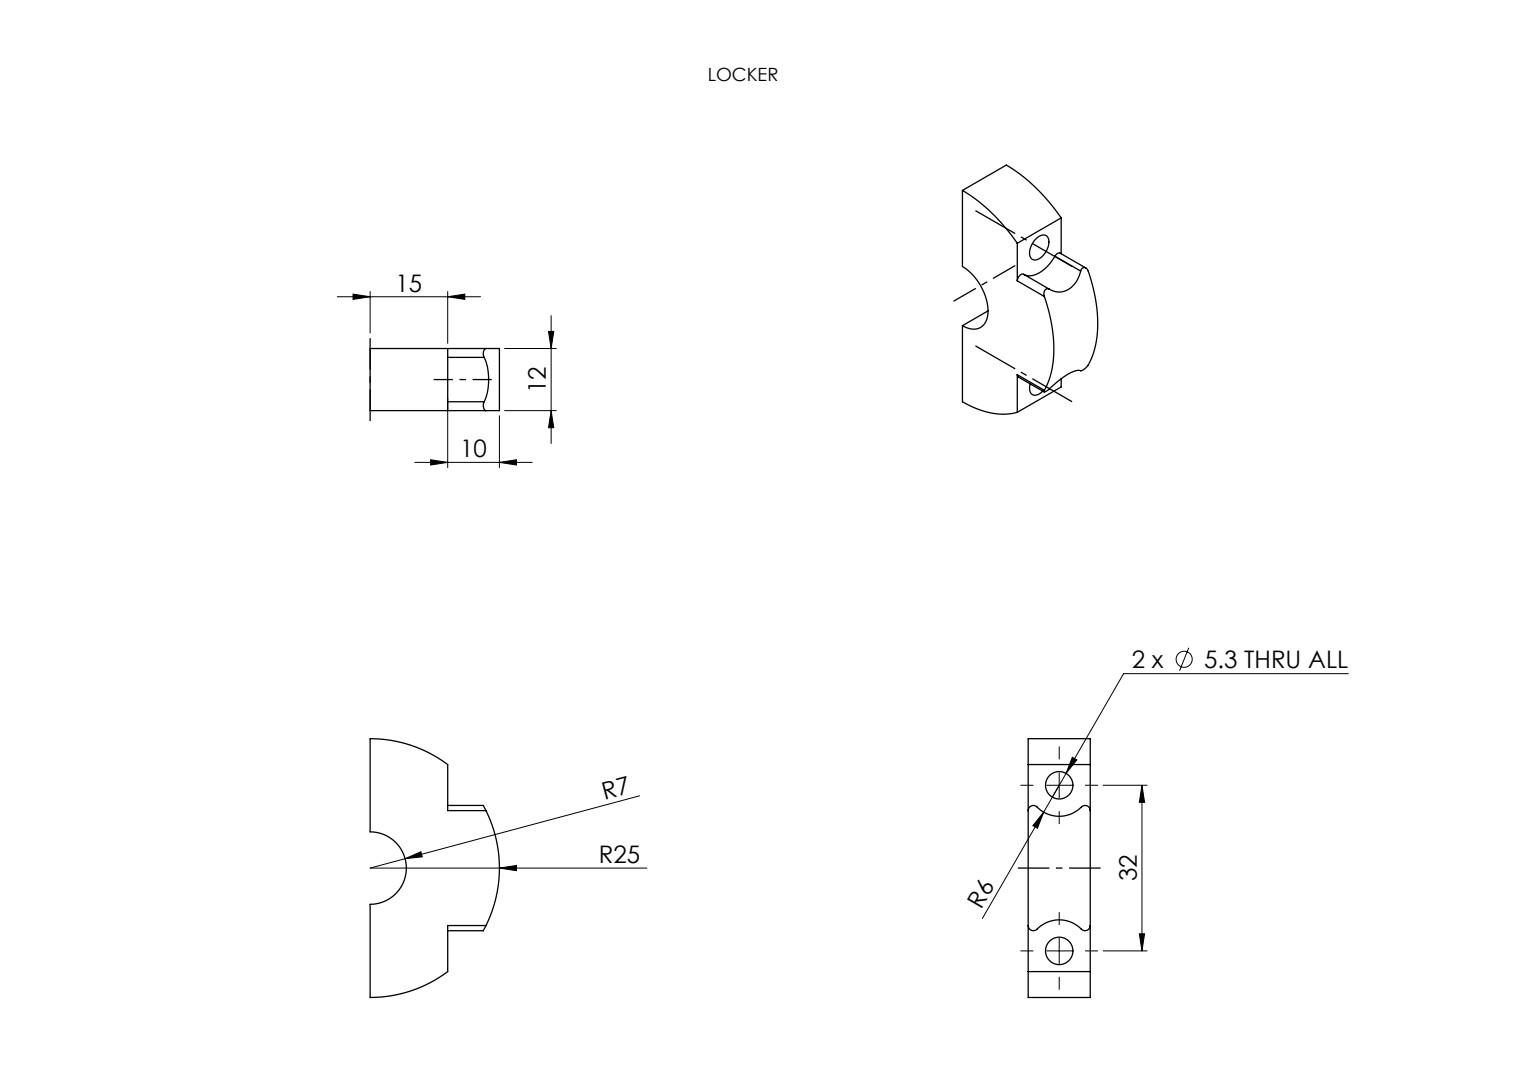
ISO-10303-21;
HEADER;
FILE_DESCRIPTION (('STEP AP214'),
    '1' );
FILE_NAME ('locker.step',
    '2026-10-08T14:09:18',
    ( '' ),
    ( '' ),
    'SwSTEP 2.0',
    'SolidWorks 2026',
    '' );
FILE_SCHEMA (( 'AUTOMOTIVE_DESIGN' ));
ENDSEC;

DATA;
#1=LINE ( 'NONE', #1937, #4329 ) ;
#6=AXIS2_PLACEMENT_3D ( 'NONE', #3174, #4687, #3807 ) ;
#21=AXIS2_PLACEMENT_3D ( 'NONE', #885, #4593, #1214 ) ;
#23=ORIENTED_EDGE ( 'NONE', *, *, #1515, .T. ) ;
#25=CARTESIAN_POINT ( 'NONE',  ( 22.89074894326665088, 10.05057747304974924, -26.80355754512474675 ) ) ;
#32=CARTESIAN_POINT ( 'NONE',  ( 15.00000000000000178, -16.00000000000000000, -26.00000000000000355 ) ) ;
#39=DIRECTION ( 'NONE',  ( 0.000000000000000000, 0.000000000000000000, -1.000000000000000000 ) ) ;
#60=ORIENTED_EDGE ( 'NONE', *, *, #3152, .T. ) ;
#64=DIRECTION ( 'NONE',  ( 0.000000000000000000, -1.000000000000000000, 0.000000000000000000 ) ) ;
#67=CARTESIAN_POINT ( 'NONE',  ( 25.00000000000000000, -11.80087472665741011, -21.71428571428571530 ) ) ;
#72=CARTESIAN_POINT ( 'NONE',  ( 22.90859662698202470, -10.00982993400317334, -25.60100662543646877 ) ) ;
#79=DIRECTION ( 'NONE',  ( 1.000000000000000000, 0.000000000000000000, 0.000000000000000000 ) ) ;
#81=CARTESIAN_POINT ( 'NONE',  ( 21.90226041726126383, 12.05376714070078847, -31.32044994803182547 ) ) ;
#88=CARTESIAN_POINT ( 'NONE',  ( 15.00000000000000000, 11.10102051443364424, -21.00000000000000000 ) ) ;
#101=AXIS2_PLACEMENT_3D ( 'NONE', #4841, #1750, #2213 ) ;
#104=CARTESIAN_POINT ( 'NONE',  ( 22.03949535914419755, -11.80087472665740655, -21.71428571428571885 ) ) ;
#113=EDGE_CURVE ( 'NONE', #181, #2456, #4183, .T. ) ;
#114=ORIENTED_EDGE ( 'NONE', *, *, #457, .T. ) ;
#122=CIRCLE ( 'NONE', #3524, 2.649999999999995914 ) ;
#129=EDGE_LOOP ( 'NONE', ( #232, #1337, #3287, #640, #1099, #3548 ) ) ;
#133=EDGE_CURVE ( 'NONE', #4849, #2456, #528, .T. ) ;
#139=SURFACE_STYLE_USAGE ( .BOTH. , #2050 ) ;
#141=CYLINDRICAL_SURFACE ( 'NONE', #2344, 2.649999999999992806 ) ;
#145=CARTESIAN_POINT ( 'NONE',  ( 25.00000000000000000, 11.80087472665740478, -30.28571428571428470 ) ) ;
#155=CARTESIAN_POINT ( 'NONE',  ( 15.00000000000000000, 16.00000000000000000, -26.00000000000000355 ) ) ;
#156=CARTESIAN_POINT ( 'NONE',  ( 22.03949535914419755, -11.80087472665740655, -21.71428571428571885 ) ) ;
#159=B_SPLINE_CURVE_WITH_KNOTS ( 'NONE', 3,
 ( #3123, #2291, #1168, #2640, #4187, #3835, #3809, #759, #1888, #81, #4617, #385, #2749, #3439, #2697, #3415 ),
 .UNSPECIFIED., .F., .F.,
 ( 4, 2, 2, 2, 2, 2, 2, 4 ),
 ( 0.000000000000000000, 0.0003092645584586380158, 0.0006185291169172760315, 0.0009277936753759139388, 0.001237058233834552063, 0.001546322792293189970, 0.001855587350751827878, 0.002474116467669114968 ),
 .UNSPECIFIED. ) ;
#160=ORIENTED_EDGE ( 'NONE', *, *, #457, .F. ) ;
#162=CARTESIAN_POINT ( 'NONE',  ( 22.40016391766193138, 11.10102051443364424, -20.00000000000000000 ) ) ;
#165=VERTEX_POINT ( 'NONE', #2693 ) ;
#180=ORIENTED_EDGE ( 'NONE', *, *, #1366, .T. ) ;
#181=VERTEX_POINT ( 'NONE', #4357 ) ;
#184=AXIS2_PLACEMENT_3D ( 'NONE', #4270, #4673, #3105 ) ;
#190=B_SPLINE_CURVE_WITH_KNOTS ( 'NONE', 3,
 ( #2928, #244, #278, #4394, #4375, #967, #201, #1739, #4801, #3276 ),
 .UNSPECIFIED., .F., .F.,
 ( 4, 2, 2, 2, 4 ),
 ( 0.000000000000000000, 0.0006190800217238748033, 0.001238160043447749607, 0.001857240065171624410, 0.002476320086895499213 ),
 .UNSPECIFIED. ) ;
#191=VECTOR ( 'NONE', #2924, 1000.000000000000000 ) ;
#193=SURFACE_STYLE_FILL_AREA ( #525 ) ;
#201=CARTESIAN_POINT ( 'NONE',  ( 22.04417985544613146, -11.79351823160729751, -31.74594383812769749 ) ) ;
#213=CARTESIAN_POINT ( 'NONE',  ( 0.000000000000000000, -25.00000000000000000, -20.00000000000000000 ) ) ;
#221=CARTESIAN_POINT ( 'NONE',  ( 25.00000000000000000, 11.10102051443364424, -21.00000000000000000 ) ) ;
#229=CARTESIAN_POINT ( 'NONE',  ( 0.000000000000000000, 0.000000000000000000, -32.00000000000000000 ) ) ;
#230=FACE_OUTER_BOUND ( 'NONE', #3929, .T. ) ;
#232=ORIENTED_EDGE ( 'NONE', *, *, #1612, .F. ) ;
#244=CARTESIAN_POINT ( 'NONE',  ( 21.96482728828171460, -11.94032596560094461, -30.42234803747852467 ) ) ;
#260=DIRECTION ( 'NONE',  ( 1.000000000000000000, -0.000000000000000000, -0.000000000000000000 ) ) ;
#263=PRODUCT ( 'locker', 'locker', '', ( #3647 ) ) ;
#266=VECTOR ( 'NONE', #64, 1000.000000000000000 ) ;
#268=CIRCLE ( 'NONE', #3072, 25.00000000000000000 ) ;
#273=ORIENTED_EDGE ( 'NONE', *, *, #2286, .F. ) ;
#278=CARTESIAN_POINT ( 'NONE',  ( 21.90877321452243365, -12.04191644460182431, -30.60336459293191780 ) ) ;
#284=CARTESIAN_POINT ( 'NONE',  ( 22.76747806470418567, 10.32821797429375010, -24.00231280675427215 ) ) ;
#294=DIRECTION ( 'NONE',  ( 0.000000000000000000, 0.000000000000000000, -1.000000000000000000 ) ) ;
#295=ADVANCED_FACE ( 'NONE', ( #2885 ), #673, .T. ) ;
#298=B_SPLINE_CURVE_WITH_KNOTS ( 'NONE', 3,
 ( #2171, #3292, #3229, #3661, #2073, #4458, #3590, #4061, #2542, #162 ),
 .UNSPECIFIED., .F., .F.,
 ( 4, 2, 2, 2, 4 ),
 ( 0.000000000000000000, 0.0006190800217238756707, 0.001238160043447751341, 0.001857240065171627012, 0.002476320086895502683 ),
 .UNSPECIFIED. ) ;
#307=DIRECTION ( 'NONE',  ( 0.000000000000000000, 0.000000000000000000, -1.000000000000000000 ) ) ;
#310=DIRECTION ( 'NONE',  ( 0.000000000000000000, 1.000000000000000000, 0.000000000000000000 ) ) ;
#318=VERTEX_POINT ( 'NONE', #4781 ) ;
#343=MECHANICAL_DESIGN_GEOMETRIC_PRESENTATION_REPRESENTATION('',(#3776),#4337);
#347=( NAMED_UNIT ( * ) PLANE_ANGLE_UNIT ( ) SI_UNIT ( $, .RADIAN. ) );
#364=DIRECTION ( 'NONE',  ( 0.000000000000000000, 0.000000000000000000, -1.000000000000000000 ) ) ;
#371=ORIENTED_EDGE ( 'NONE', *, *, #1787, .F. ) ;
#375=CARTESIAN_POINT ( 'NONE',  ( 22.61674500023159240, -10.65336738338371347, -28.73004557699725936 ) ) ;
#376=PLANE ( 'NONE',  #1226 ) ;
#381=ADVANCED_FACE ( 'NONE', ( #1705 ), #3239, .T. ) ;
#385=CARTESIAN_POINT ( 'NONE',  ( 21.87320774003120150, 12.10631999347636167, -31.01543084472370992 ) ) ;
#390=LINE ( 'NONE', #1915, #2331 ) ;
#393=UNCERTAINTY_MEASURE_WITH_UNIT (LENGTH_MEASURE( 1.000000000000000082E-05 ), #500, 'distance_accuracy_value', 'NONE');
#394=CARTESIAN_POINT ( 'NONE',  ( 15.00000000000000000, 11.10102051443364424, -20.00000000000000000 ) ) ;
#395=CARTESIAN_POINT ( 'NONE',  ( -3.642919299551294898E-14, -16.00000000000000000, -26.00000000000000355 ) ) ;
#400=EDGE_CURVE ( 'NONE', #2569, #4849, #4958, .T. ) ;
#402=DIRECTION ( 'NONE',  ( 1.000000000000000000, 2.036697447658493800E-15, 0.000000000000000000 ) ) ;
#427=CIRCLE ( 'NONE', #3306, 2.649999999999985700 ) ;
#429=CARTESIAN_POINT ( 'NONE',  ( 0.000000000000000000, 0.000000000000000000, -32.00000000000000000 ) ) ;
#437=CARTESIAN_POINT ( 'NONE',  ( 22.66008913276283820, 10.56067522606771547, -28.54043899563736986 ) ) ;
#457=EDGE_CURVE ( 'NONE', #181, #2569, #122, .T. ) ;
#464=CARTESIAN_POINT ( 'NONE',  ( 22.88998946896871445, 10.05230818559221539, -25.18361442742383360 ) ) ;
#472=CARTESIAN_POINT ( 'NONE',  ( 21.87533763385574659, -12.10248395817102107, -21.08882388928228835 ) ) ;
#485=PRODUCT_DEFINITION_CONTEXT ( 'detailed design', #2667, 'design' ) ;
#486=CARTESIAN_POINT ( 'NONE',  ( 22.31344532614783205, -11.27701289969359522, -22.27898711539451071 ) ) ;
#489=EDGE_CURVE ( 'NONE', #3217, #2692, #1229, .T. ) ;
#492=SHAPE_DEFINITION_REPRESENTATION ( #1211, #4221 ) ;
#500=( LENGTH_UNIT ( ) NAMED_UNIT ( * ) SI_UNIT ( .MILLI., .METRE. ) );
#503=AXIS2_PLACEMENT_3D ( 'NONE', #890, #2321, #39 ) ;
#510=VECTOR ( 'NONE', #740, 1000.000000000000000 ) ;
#512=ORIENTED_EDGE ( 'NONE', *, *, #1917, .T. ) ;
#516=DIRECTION ( 'NONE',  ( 1.000000000000000000, -0.000000000000000000, -0.000000000000000000 ) ) ;
#522=DIRECTION ( 'NONE',  ( 1.000000000000000000, -0.000000000000000000, -0.000000000000000000 ) ) ;
#525=FILL_AREA_STYLE ('',( #2096 ) ) ;
#528=CIRCLE ( 'NONE', #4589, 2.649999999999985700 ) ;
#563=ORIENTED_EDGE ( 'NONE', *, *, #3713, .T. ) ;
#580=COLOUR_RGB ( '', 0.72549020, 0.75294118, 0.79215686) ;
#586=VERTEX_POINT ( 'NONE', #1997 ) ;
#588=DIRECTION ( 'NONE',  ( 0.000000000000000000, 0.000000000000000000, 1.000000000000000000 ) ) ;
#599=DIRECTION ( 'NONE',  ( -1.000000000000000000, 0.000000000000000000, 0.000000000000000000 ) ) ;
#603=DIRECTION ( 'NONE',  ( -1.000000000000000000, 0.000000000000000000, 0.000000000000000000 ) ) ;
#604=CARTESIAN_POINT ( 'NONE',  ( 15.00000000000000000, -11.80087472665740655, -21.71428571428571885 ) ) ;
#612=EDGE_LOOP ( 'NONE', ( #60, #1655 ) ) ;
#617=MECHANICAL_DESIGN_GEOMETRIC_PRESENTATION_REPRESENTATION('',(#1267),#2875);
#618=DIRECTION ( 'NONE',  ( -0.000000000000000000, -0.000000000000000000, 1.000000000000000000 ) ) ;
#620=PRESENTATION_STYLE_ASSIGNMENT (( #4050 ) ) ;
#628=EDGE_CURVE ( 'NONE', #4218, #3494, #3207, .T. ) ;
#636=FACE_BOUND ( 'NONE', #612, .T. ) ;
#640=ORIENTED_EDGE ( 'NONE', *, *, #4116, .T. ) ;
#649=CYLINDRICAL_SURFACE ( 'NONE', #973, 6.999999999999999112 ) ;
#651=CIRCLE ( 'NONE', #978, 2.649999999999995914 ) ;
#668=DIRECTION ( 'NONE',  ( 1.000000000000000000, 0.000000000000000000, 0.000000000000000000 ) ) ;
#672=CARTESIAN_POINT ( 'NONE',  ( 0.000000000000000000, -25.00000000000000000, -32.00000000000000000 ) ) ;
#673=CYLINDRICAL_SURFACE ( 'NONE', #4506, 1.000000000000000888 ) ;
#684=EDGE_CURVE ( 'NONE', #2597, #4218, #190, .T. ) ;
#688=LINE ( 'NONE', #3368, #510 ) ;
#693=ORIENTED_EDGE ( 'NONE', *, *, #4446, .T. ) ;
#696=CARTESIAN_POINT ( 'NONE',  ( 0.000000000000000000, 0.000000000000000000, -20.00000000000000000 ) ) ;
#698=CARTESIAN_POINT ( 'NONE',  ( 2.444036937190193033E-14, 6.999999999999999112, -20.00000000000000000 ) ) ;
#699=FACE_BOUND ( 'NONE', #2377, .T. ) ;
#705=CARTESIAN_POINT ( 'NONE',  ( 0.000000000000000000, 25.00000000000000000, -32.00000000000000000 ) ) ;
#710=DIRECTION ( 'NONE',  ( 0.000000000000000000, 0.000000000000000000, 1.000000000000000000 ) ) ;
#719=ADVANCED_FACE ( 'NONE', ( #2078 ), #1718, .F. ) ;
#730=DIRECTION ( 'NONE',  ( 0.000000000000000000, 0.000000000000000000, -1.000000000000000000 ) ) ;
#740=DIRECTION ( 'NONE',  ( -2.036697447658493800E-15, 1.000000000000000000, 0.000000000000000000 ) ) ;
#746=EDGE_CURVE ( 'NONE', #2092, #2240, #994, .T. ) ;
#748=CARTESIAN_POINT ( 'NONE',  ( 22.31144310522464735, -11.28096319364321509, -29.72586080439007006 ) ) ;
#749=EDGE_CURVE ( 'NONE', #1695, #3657, #3997, .T. ) ;
#755=ADVANCED_BREP_SHAPE_REPRESENTATION ( '', ( #2079, #1918 ), #1581 ) ;
#759=CARTESIAN_POINT ( 'NONE',  ( 21.97815564317848924, 11.91494984865602191, -31.58906108478248953 ) ) ;
#781=CARTESIAN_POINT ( 'NONE',  ( 22.04753367391286645, -11.78607713658132994, -20.26503649943386876 ) ) ;
#787=FILL_AREA_STYLE ('',( #1511 ) ) ;
#796=VECTOR ( 'NONE', #2151, 1000.000000000000000 ) ;
#797=CARTESIAN_POINT ( 'NONE',  ( 22.87614623887219167, 10.08384657499285808, -24.98007506026046798 ) ) ;
#801=AXIS2_PLACEMENT_3D ( 'NONE', #2152, #4779, #1345 ) ;
#807=CARTESIAN_POINT ( 'NONE',  ( 21.88691174701116182, -12.08152700620045117, -20.77757659040560512 ) ) ;
#810=CIRCLE ( 'NONE', #1521, 2.649999999999985700 ) ;
#821=ORIENTED_EDGE ( 'NONE', *, *, #3902, .T. ) ;
#827=ORIENTED_EDGE ( 'NONE', *, *, #2659, .T. ) ;
#831=CARTESIAN_POINT ( 'NONE',  ( 22.91733099102425442, 9.989778831080645460, -25.99421712970024245 ) ) ;
#833=DIRECTION ( 'NONE',  ( 0.000000000000000000, 0.000000000000000000, 1.000000000000000000 ) ) ;
#839=LINE ( 'NONE', #2341, #3531 ) ;
#840=CARTESIAN_POINT ( 'NONE',  ( 21.87320774003119794, -12.10631999347636345, -20.98456915527629363 ) ) ;
#847=ORIENTED_EDGE ( 'NONE', *, *, #133, .T. ) ;
#849=EDGE_CURVE ( 'NONE', #1731, #4866, #1094, .T. ) ;
#855=CARTESIAN_POINT ( 'NONE',  ( 22.52717933085839874, -10.84147272832753472, -22.92928814334748466 ) ) ;
#862=FACE_OUTER_BOUND ( 'NONE', #1009, .T. ) ;
#864=ORIENTED_EDGE ( 'NONE', *, *, #3599, .F. ) ;
#870=EDGE_CURVE ( 'NONE', #2692, #3603, #4723, .T. ) ;
#878=CARTESIAN_POINT ( 'NONE',  ( 15.00000000000000000, -11.10102051443364068, -32.00000000000000000 ) ) ;
#880=EDGE_CURVE ( 'NONE', #3891, #4613, #1042, .T. ) ;
#882=AXIS2_PLACEMENT_3D ( 'NONE', #3346, #4515, #1738 ) ;
#884=DIRECTION ( 'NONE',  ( 0.000000000000000000, 0.000000000000000000, -1.000000000000000000 ) ) ;
#885=CARTESIAN_POINT ( 'NONE',  ( 25.00000000000000000, -11.10102051443364424, -21.00000000000000000 ) ) ;
#890=CARTESIAN_POINT ( 'NONE',  ( 15.00000000000000000, 11.10102051443364068, -31.00000000000000000 ) ) ;
#892=AXIS2_PLACEMENT_3D ( 'NONE', #2942, #989, #2146 ) ;
#916=DIRECTION ( 'NONE',  ( 0.000000000000000000, 0.000000000000000000, -1.000000000000000000 ) ) ;
#918=CARTESIAN_POINT ( 'NONE',  ( 25.00000000000000000, 11.10102051443364068, -31.00000000000000000 ) ) ;
#924=VECTOR ( 'NONE', #3089, 1000.000000000000000 ) ;
#929=ORIENTED_EDGE ( 'NONE', *, *, #746, .F. ) ;
#932=LINE ( 'NONE', #3978, #3232 ) ;
#935=CARTESIAN_POINT ( 'NONE',  ( 0.000000000000000000, 0.000000000000000000, -20.00000000000000000 ) ) ;
#942=LINE ( 'NONE', #213, #4561 ) ;
#943=CARTESIAN_POINT ( 'NONE',  ( 25.00000000000000000, 0.000000000000000000, -20.00000000000000000 ) ) ;
#959=ORIENTED_EDGE ( 'NONE', *, *, #3343, .T. ) ;
#963=EDGE_CURVE ( 'NONE', #1731, #3126, #1842, .T. ) ;
#965=DIRECTION ( 'NONE',  ( 1.000000000000000000, 0.000000000000000000, 0.000000000000000000 ) ) ;
#966=EDGE_CURVE ( 'NONE', #4690, #2597, #390, .T. ) ;
#967=CARTESIAN_POINT ( 'NONE',  ( 21.97031423931356287, -11.92955703141274881, -31.59565500209243183 ) ) ;
#973=AXIS2_PLACEMENT_3D ( 'NONE', #3359, #2664, #1028 ) ;
#978=AXIS2_PLACEMENT_3D ( 'NONE', #2150, #2475, #2105 ) ;
#985=ORIENTED_EDGE ( 'NONE', *, *, #2110, .T. ) ;
#987=VERTEX_POINT ( 'NONE', #1248 ) ;
#989=DIRECTION ( 'NONE',  ( 1.000000000000000000, -0.000000000000000000, -0.000000000000000000 ) ) ;
#992=CARTESIAN_POINT ( 'NONE',  ( 15.00000000000000000, -20.00000000000000355, -32.00000000000000000 ) ) ;
#994=LINE ( 'NONE', #2477, #4000 ) ;
#1009=EDGE_LOOP ( 'NONE', ( #3602, #4092, #2424, #2514 ) ) ;
#1024=VERTEX_POINT ( 'NONE', #4598 ) ;
#1026=CARTESIAN_POINT ( 'NONE',  ( 22.52496067886514197, 10.84608396733234592, -22.92156229269478374 ) ) ;
#1028=DIRECTION ( 'NONE',  ( 1.000000000000000000, 0.000000000000000000, 0.000000000000000000 ) ) ;
#1036=ORIENTED_EDGE ( 'NONE', *, *, #4737, .T. ) ;
#1042=LINE ( 'NONE', #3766, #4728 ) ;
#1060=EDGE_CURVE ( 'NONE', #3126, #4359, #2094, .T. ) ;
#1067=VERTEX_POINT ( 'NONE', #1221 ) ;
#1069=CARTESIAN_POINT ( 'NONE',  ( 22.03949535914419755, -11.80087472665740655, -21.71428571428571885 ) ) ;
#1081=CARTESIAN_POINT ( 'NONE',  ( 22.40016391766193493, 11.10102051443364068, -32.00000000000000000 ) ) ;
#1094=LINE ( 'NONE', #3399, #2408 ) ;
#1096=ORIENTED_EDGE ( 'NONE', *, *, #3247, .T. ) ;
#1099=ORIENTED_EDGE ( 'NONE', *, *, #1951, .F. ) ;
#1115=DIRECTION ( 'NONE',  ( 1.000000000000000000, 0.000000000000000000, 0.000000000000000000 ) ) ;
#1143=VECTOR ( 'NONE', #4180, 1000.000000000000000 ) ;
#1145=FACE_OUTER_BOUND ( 'NONE', #2865, .T. ) ;
#1146=CARTESIAN_POINT ( 'NONE',  ( 0.000000000000000000, 0.000000000000000000, 0.000000000000000000 ) ) ;
#1147=CARTESIAN_POINT ( 'NONE',  ( 15.00000000000000000, 16.00000000000000000, -26.00000000000000355 ) ) ;
#1158=CARTESIAN_POINT ( 'NONE',  ( 22.76902711785762534, -10.32479573876449486, -24.01193718893786411 ) ) ;
#1163=EDGE_LOOP ( 'NONE', ( #929, #3191, #2786, #3592, #1633, #1962 ) ) ;
#1164=DIRECTION ( 'NONE',  ( 1.000000000000000000, -0.000000000000000000, -0.000000000000000000 ) ) ;
#1168=CARTESIAN_POINT ( 'NONE',  ( 22.30769810302473388, 11.28612666381332730, -31.98709346889334881 ) ) ;
#1174=ORIENTED_EDGE ( 'NONE', *, *, #4886, .F. ) ;
#1192=CARTESIAN_POINT ( 'NONE',  ( 22.21646894734064759, -11.46466559648295558, -20.06384827235568835 ) ) ;
#1206=CARTESIAN_POINT ( 'NONE',  ( 22.18526740102420547, -11.52862861652370441, -30.01896866400023356 ) ) ;
#1211=PRODUCT_DEFINITION_SHAPE ( 'NONE', 'NONE',  #2072 ) ;
#1214=DIRECTION ( 'NONE',  ( 0.000000000000000000, 0.000000000000000000, 1.000000000000000000 ) ) ;
#1219=( NAMED_UNIT ( * ) SI_UNIT ( $, .STERADIAN. ) SOLID_ANGLE_UNIT ( ) );
#1221=CARTESIAN_POINT ( 'NONE',  ( 0.000000000000000000, 25.00000000000000000, -32.00000000000000000 ) ) ;
#1224=LINE ( 'NONE', #3520, #266 ) ;
#1225=EDGE_LOOP ( 'NONE', ( #3596, #4059, #4019, #985 ) ) ;
#1226=AXIS2_PLACEMENT_3D ( 'NONE', #1449, #402, #1496 ) ;
#1229=LINE ( 'NONE', #67, #4473 ) ;
#1230=AXIS2_PLACEMENT_3D ( 'NONE', #88, #1590, #4909 ) ;
#1232=ORIENTED_EDGE ( 'NONE', *, *, #1612, .T. ) ;
#1234=CARTESIAN_POINT ( 'NONE',  ( 22.66008913276283110, -10.56067522606771547, -23.45956100436263725 ) ) ;
#1241=DIRECTION ( 'NONE',  ( 1.000000000000000000, -0.000000000000000000, -0.000000000000000000 ) ) ;
#1242=EDGE_CURVE ( 'NONE', #2366, #165, #942, .T. ) ;
#1247=ORIENTED_EDGE ( 'NONE', *, *, #1242, .T. ) ;
#1248=CARTESIAN_POINT ( 'NONE',  ( 6.999999999999999112, 0.000000000000000000, -32.00000000000000000 ) ) ;
#1258=EDGE_LOOP ( 'NONE', ( #1815, #3183, #2999, #3488 ) ) ;
#1267=STYLED_ITEM ( 'NONE', ( #1990 ), #755 ) ;
#1269=( NAMED_UNIT ( * ) PLANE_ANGLE_UNIT ( ) SI_UNIT ( $, .RADIAN. ) );
#1274=CYLINDRICAL_SURFACE ( 'NONE', #4467, 25.00000000000000000 ) ;
#1276=ORIENTED_EDGE ( 'NONE', *, *, #4303, .T. ) ;
#1286=DIRECTION ( 'NONE',  ( -1.000000000000000000, 0.000000000000000000, 0.000000000000000000 ) ) ;
#1297=CIRCLE ( 'NONE', #3372, 25.00000000000000000 ) ;
#1300=AXIS2_PLACEMENT_3D ( 'NONE', #229, #4403, #603 ) ;
#1303=CIRCLE ( 'NONE', #2022, 2.649999999999995914 ) ;
#1307=VECTOR ( 'NONE', #2791, 1000.000000000000000 ) ;
#1312=EDGE_LOOP ( 'NONE', ( #3317, #1232, #2731, #3928, #2819, #959, #2054, #4784, #3946, #4335, #3757, #4091 ) ) ;
#1322=FACE_OUTER_BOUND ( 'NONE', #2719, .T. ) ;
#1337=ORIENTED_EDGE ( 'NONE', *, *, #746, .T. ) ;
#1345=DIRECTION ( 'NONE',  ( 0.000000000000000000, 0.000000000000000000, -1.000000000000000000 ) ) ;
#1366=EDGE_CURVE ( 'NONE', #4359, #318, #4531, .T. ) ;
#1370=LINE ( 'NONE', #672, #4067 ) ;
#1396=EDGE_CURVE ( 'NONE', #586, #3657, #2656, .T. ) ;
#1408=CYLINDRICAL_SURFACE ( 'NONE', #3219, 1.000000000000000888 ) ;
#1413=DIRECTION ( 'NONE',  ( 1.000000000000000000, 0.000000000000000000, 0.000000000000000000 ) ) ;
#1424=LINE ( 'NONE', #3707, #2981 ) ;
#1434=DIRECTION ( 'NONE',  ( -1.000000000000000000, -0.000000000000000000, -0.000000000000000000 ) ) ;
#1445=ADVANCED_FACE ( 'NONE', ( #2672 ), #1481, .F. ) ;
#1446=CIRCLE ( 'NONE', #1300, 6.999999999999999112 ) ;
#1449=CARTESIAN_POINT ( 'NONE',  ( 0.000000000000000000, -25.00000000000000000, -32.00000000000000000 ) ) ;
#1466=CARTESIAN_POINT ( 'NONE',  ( 25.00000000000000000, 0.000000000000000000, -32.00000000000000000 ) ) ;
#1472=ORIENTED_EDGE ( 'NONE', *, *, #4303, .F. ) ;
#1475=FACE_OUTER_BOUND ( 'NONE', #3274, .T. ) ;
#1478=EDGE_CURVE ( 'NONE', #1067, #318, #1297, .T. ) ;
#1481=PLANE ( 'NONE',  #2574 ) ;
#1490=UNCERTAINTY_MEASURE_WITH_UNIT (LENGTH_MEASURE( 1.000000000000000082E-05 ), #4932, 'distance_accuracy_value', 'NONE');
#1496=DIRECTION ( 'NONE',  ( -2.036697447658493800E-15, 1.000000000000000000, 0.000000000000000000 ) ) ;
#1508=ADVANCED_FACE ( 'NONE', ( #3912 ), #3833, .F. ) ;
#1511=FILL_AREA_STYLE_COLOUR ( '', #580 ) ;
#1515=EDGE_CURVE ( 'NONE', #318, #4003, #1, .T. ) ;
#1521=AXIS2_PLACEMENT_3D ( 'NONE', #32, #1241, #3099 ) ;
#1534=CARTESIAN_POINT ( 'NONE',  ( 22.40016391766193138, -11.10102051443364424, -20.00000000000000000 ) ) ;
#1535=ORIENTED_EDGE ( 'NONE', *, *, #3247, .F. ) ;
#1539=EDGE_LOOP ( 'NONE', ( #3461, #1174, #3112, #4718 ) ) ;
#1544=EDGE_CURVE ( 'NONE', #2456, #4849, #810, .T. ) ;
#1554=CARTESIAN_POINT ( 'NONE',  ( 22.47483654244695472, -10.94974330264383156, -29.24541893584931529 ) ) ;
#1573=CARTESIAN_POINT ( 'NONE',  ( 22.03949535914419755, -11.80087472665740478, -30.28571428571428470 ) ) ;
#1581=( GEOMETRIC_REPRESENTATION_CONTEXT ( 3 ) GLOBAL_UNCERTAINTY_ASSIGNED_CONTEXT ( ( #393 ) ) GLOBAL_UNIT_ASSIGNED_CONTEXT ( ( #500, #1269, #2858 ) ) REPRESENTATION_CONTEXT ( 'NONE', 'WORKASPACE' ) );
#1590=DIRECTION ( 'NONE',  ( -1.000000000000000000, -0.000000000000000000, -0.000000000000000000 ) ) ;
#1597=CARTESIAN_POINT ( 'NONE',  ( 22.87614623887219523, -10.08384657499285808, -27.01992493973954623 ) ) ;
#1598=DIRECTION ( 'NONE',  ( -1.357798298438996130E-15, 1.000000000000000000, 0.000000000000000000 ) ) ;
#1608=CARTESIAN_POINT ( 'NONE',  ( 22.40016391766193493, -11.10102051443364068, -32.00000000000000000 ) ) ;
#1611=ORIENTED_EDGE ( 'NONE', *, *, #113, .T. ) ;
#1612=EDGE_CURVE ( 'NONE', #2092, #4218, #3063, .T. ) ;
#1624=DIRECTION ( 'NONE',  ( -1.000000000000000000, 0.000000000000000000, 0.000000000000000000 ) ) ;
#1628=DIRECTION ( 'NONE',  ( 1.000000000000000000, -0.000000000000000000, -0.000000000000000000 ) ) ;
#1633=ORIENTED_EDGE ( 'NONE', *, *, #2286, .T. ) ;
#1636=DIRECTION ( 'NONE',  ( 0.000000000000000000, 0.000000000000000000, -1.000000000000000000 ) ) ;
#1646=ORIENTED_EDGE ( 'NONE', *, *, #400, .T. ) ;
#1652=DIRECTION ( 'NONE',  ( 0.000000000000000000, 0.000000000000000000, -1.000000000000000000 ) ) ;
#1655=ORIENTED_EDGE ( 'NONE', *, *, #3196, .T. ) ;
#1656=ORIENTED_EDGE ( 'NONE', *, *, #3717, .T. ) ;
#1670=DIRECTION ( 'NONE',  ( -0.000000000000000000, -0.000000000000000000, 1.000000000000000000 ) ) ;
#1673=EDGE_CURVE ( 'NONE', #2240, #4310, #2429, .T. ) ;
#1688=SHAPE_REPRESENTATION_RELATIONSHIP ( 'NONE' , 'NONE' ,  #4221, #755 ) ;
#1695=VERTEX_POINT ( 'NONE', #3246 ) ;
#1700=AXIS2_PLACEMENT_3D ( 'NONE', #918, #2142, #4815 ) ;
#1703=EDGE_CURVE ( 'NONE', #987, #3261, #1446, .T. ) ;
#1705=FACE_OUTER_BOUND ( 'NONE', #1312, .T. ) ;
#1714=CARTESIAN_POINT ( 'NONE',  ( 0.000000000000000000, 0.000000000000000000, -32.00000000000000000 ) ) ;
#1718=CYLINDRICAL_SURFACE ( 'NONE', #801, 2.649999999999992806 ) ;
#1728=DIRECTION ( 'NONE',  ( 1.000000000000000000, -0.000000000000000000, -0.000000000000000000 ) ) ;
#1731=VERTEX_POINT ( 'NONE', #4712 ) ;
#1738=DIRECTION ( 'NONE',  ( 0.000000000000000000, 0.000000000000000000, 1.000000000000000000 ) ) ;
#1739=CARTESIAN_POINT ( 'NONE',  ( 22.21307774062919194, -11.47223234890554266, -31.94772731936956944 ) ) ;
#1743=SURFACE_SIDE_STYLE ('',( #2322 ) ) ;
#1745=EDGE_CURVE ( 'NONE', #2165, #2366, #4250, .T. ) ;
#1750=DIRECTION ( 'NONE',  ( -0.000000000000000000, -0.000000000000000000, 1.000000000000000000 ) ) ;
#1756=CARTESIAN_POINT ( 'NONE',  ( 25.00000000000000000, -11.10102051443364068, -31.00000000000000000 ) ) ;
#1769=DIRECTION ( 'NONE',  ( -0.000000000000000000, -0.000000000000000000, 1.000000000000000000 ) ) ;
#1787=EDGE_CURVE ( 'NONE', #1889, #2416, #3385, .T. ) ;
#1801=CYLINDRICAL_SURFACE ( 'NONE', #2637, 25.00000000000000000 ) ;
#1805=CARTESIAN_POINT ( 'NONE',  ( 22.82142399877221095, 10.20738559227135944, -24.38442231784400249 ) ) ;
#1811=DIRECTION ( 'NONE',  ( -1.000000000000000000, 0.000000000000000000, -0.000000000000000000 ) ) ;
#1812=DIRECTION ( 'NONE',  ( 0.000000000000000000, 0.000000000000000000, -1.000000000000000000 ) ) ;
#1813=ORIENTED_EDGE ( 'NONE', *, *, #849, .F. ) ;
#1815=ORIENTED_EDGE ( 'NONE', *, *, #3196, .F. ) ;
#1816=DIRECTION ( 'NONE',  ( -1.357798298438996130E-15, 1.000000000000000000, 0.000000000000000000 ) ) ;
#1817=CYLINDRICAL_SURFACE ( 'NONE', #882, 5.999999999999998224 ) ;
#1828=ORIENTED_EDGE ( 'NONE', *, *, #2472, .F. ) ;
#1829=AXIS2_PLACEMENT_3D ( 'NONE', #429, #4625, #2380 ) ;
#1835=PLANE ( 'NONE',  #3774 ) ;
#1842=CIRCLE ( 'NONE', #4646, 5.999999999999998224 ) ;
#1843=LINE ( 'NONE', #4804, #3994 ) ;
#1846=ADVANCED_FACE ( 'NONE', ( #3335 ), #2631, .F. ) ;
#1864=ORIENTED_EDGE ( 'NONE', *, *, #1396, .F. ) ;
#1867=DIRECTION ( 'NONE',  ( 1.000000000000000000, -0.000000000000000000, -0.000000000000000000 ) ) ;
#1875=VERTEX_POINT ( 'NONE', #3406 ) ;
#1878=CARTESIAN_POINT ( 'NONE',  ( 22.31144310522464735, 11.28096319364322042, -22.27413919560993705 ) ) ;
#1886=DIRECTION ( 'NONE',  ( -1.000000000000000000, 0.000000000000000000, 0.000000000000000000 ) ) ;
#1888=CARTESIAN_POINT ( 'NONE',  ( 21.94848156259736527, 11.96939725984945113, -31.50629648535032601 ) ) ;
#1889=VERTEX_POINT ( 'NONE', #698 ) ;
#1899=ORIENTED_EDGE ( 'NONE', *, *, #966, .F. ) ;
#1915=CARTESIAN_POINT ( 'NONE',  ( 25.00000000000000000, -11.80087472665740478, -30.28571428571428470 ) ) ;
#1917=EDGE_CURVE ( 'NONE', #4866, #4838, #2755, .T. ) ;
#1918=AXIS2_PLACEMENT_3D ( 'NONE', #1146, #2700, #1115 ) ;
#1921=DIRECTION ( 'NONE',  ( 1.000000000000000000, -0.000000000000000000, -0.000000000000000000 ) ) ;
#1937=CARTESIAN_POINT ( 'NONE',  ( 15.00000000000000000, 20.00000000000000355, -32.00000000000000000 ) ) ;
#1947=CARTESIAN_POINT ( 'NONE',  ( 15.00000000000000000, -20.00000000000000355, -20.00000000000000000 ) ) ;
#1951=EDGE_CURVE ( 'NONE', #2597, #3217, #2035, .T. ) ;
#1957=ORIENTED_EDGE ( 'NONE', *, *, #3902, .F. ) ;
#1959=CARTESIAN_POINT ( 'NONE',  ( 22.18564505841181855, 11.52792329777113345, -30.01827759558031161 ) ) ;
#1962=ORIENTED_EDGE ( 'NONE', *, *, #3675, .T. ) ;
#1965=DIRECTION ( 'NONE',  ( -0.000000000000000000, -0.000000000000000000, 1.000000000000000000 ) ) ;
#1972=ORIENTED_EDGE ( 'NONE', *, *, #133, .F. ) ;
#1979=CARTESIAN_POINT ( 'NONE',  ( 22.31344532614782850, 11.27701289969359166, -29.72101288460549284 ) ) ;
#1987=CARTESIAN_POINT ( 'NONE',  ( 21.94848156259736527, -11.96939725984945468, -20.49370351464968465 ) ) ;
#1988=ORIENTED_EDGE ( 'NONE', *, *, #3262, .F. ) ;
#1990=PRESENTATION_STYLE_ASSIGNMENT (( #139 ) ) ;
#1997=CARTESIAN_POINT ( 'NONE',  ( 15.00000000000000178, 16.00000000000000000, -23.35000000000001563 ) ) ;
#2004=CARTESIAN_POINT ( 'NONE',  ( 22.61871848390502393, -10.64917431867735154, -23.27817350896996018 ) ) ;
#2021=( LENGTH_UNIT ( ) NAMED_UNIT ( * ) SI_UNIT ( .MILLI., .METRE. ) );
#2022=AXIS2_PLACEMENT_3D ( 'NONE', #3650, #516, #2040 ) ;
#2035=B_SPLINE_CURVE_WITH_KNOTS ( 'NONE', 3,
 ( #1573, #1206, #748, #1554, #3504, #375, #3429, #4836, #4222, #1597, #3067, #2736, #2363, #72, #3138, #4657, #4583, #1158, #1234, #2004, #855, #2767, #486, #3532, #104 ),
 .UNSPECIFIED., .F., .F.,
 ( 4, 2, 2, 2, 2, 2, 1, 2, 2, 2, 2, 2, 4 ),
 ( 0.005424949174462418561, 0.006631086198200497259, 0.007234154710069534006, 0.007837223221938570752, 0.009043360245676652920, 0.009646428757545694871, 0.01024949726941473509, 0.01085256578128377530, 0.01145563429315281552, 0.01266177131689090810, 0.01326483982875994831, 0.01386790834062898853, 0.01507404536436706896 ),
 .UNSPECIFIED. ) ;
#2040=DIRECTION ( 'NONE',  ( 0.000000000000000000, 0.000000000000000000, -1.000000000000000000 ) ) ;
#2050=SURFACE_SIDE_STYLE ('',( #193 ) ) ;
#2054=ORIENTED_EDGE ( 'NONE', *, *, #4660, .T. ) ;
#2072=PRODUCT_DEFINITION ( 'UNKNOWN', '', #3199, #485 ) ;
#2073=CARTESIAN_POINT ( 'NONE',  ( 21.87894646962817902, 12.09631101282777621, -20.77489010396705638 ) ) ;
#2075=ORIENTED_EDGE ( 'NONE', *, *, #4563, .T. ) ;
#2078=FACE_OUTER_BOUND ( 'NONE', #2443, .T. ) ;
#2079=MANIFOLD_SOLID_BREP ( 'M5 Clearance Hole1', #4267 ) ;
#2090=CYLINDRICAL_SURFACE ( 'NONE', #3062, 2.649999999999992806 ) ;
#2092=VERTEX_POINT ( 'NONE', #1466 ) ;
#2093=ADVANCED_FACE ( 'NONE', ( #3874 ), #141, .F. ) ;
#2094=CIRCLE ( 'NONE', #503, 1.000000000000000888 ) ;
#2096=FILL_AREA_STYLE_COLOUR ( '', #4304 ) ;
#2100=AXIS2_PLACEMENT_3D ( 'NONE', #2716, #4636, #79 ) ;
#2105=DIRECTION ( 'NONE',  ( 0.000000000000000000, 0.000000000000000000, -1.000000000000000000 ) ) ;
#2110=EDGE_CURVE ( 'NONE', #2416, #4003, #4254, .T. ) ;
#2119=DIRECTION ( 'NONE',  ( -0.000000000000000000, -0.000000000000000000, 1.000000000000000000 ) ) ;
#2123=DIRECTION ( 'NONE',  ( -2.036697447658493800E-15, 1.000000000000000000, 0.000000000000000000 ) ) ;
#2129=CARTESIAN_POINT ( 'NONE',  ( 0.000000000000000000, 11.10102051443364068, -32.00000000000000000 ) ) ;
#2142=DIRECTION ( 'NONE',  ( -1.000000000000000000, 0.000000000000000000, 0.000000000000000000 ) ) ;
#2146=DIRECTION ( 'NONE',  ( 0.000000000000000000, 0.000000000000000000, -1.000000000000000000 ) ) ;
#2150=CARTESIAN_POINT ( 'NONE',  ( -3.642919299551294898E-14, 16.00000000000000000, -26.00000000000000355 ) ) ;
#2151=DIRECTION ( 'NONE',  ( 1.000000000000000000, -0.000000000000000000, -0.000000000000000000 ) ) ;
#2152=CARTESIAN_POINT ( 'NONE',  ( 15.00000000000000000, -16.00000000000000000, -26.00000000000000355 ) ) ;
#2165=VERTEX_POINT ( 'NONE', #1947 ) ;
#2171=CARTESIAN_POINT ( 'NONE',  ( 22.03949535914419400, 11.80087472665740655, -21.71428571428571885 ) ) ;
#2181=VECTOR ( 'NONE', #2211, 1000.000000000000000 ) ;
#2187=CARTESIAN_POINT ( 'NONE',  ( 22.65824501284922476, 10.56463292904780005, -23.45112747056584368 ) ) ;
#2190=CARTESIAN_POINT ( 'NONE',  ( 15.00000000000000178, 16.00000000000000000, -26.00000000000000355 ) ) ;
#2203=CARTESIAN_POINT ( 'NONE',  ( 15.00000000000000000, -11.10102051443364424, -21.00000000000000000 ) ) ;
#2204=EDGE_CURVE ( 'NONE', #2811, #2092, #268, .T. ) ;
#2207=FACE_OUTER_BOUND ( 'NONE', #129, .T. ) ;
#2210=ORIENTED_EDGE ( 'NONE', *, *, #3343, .F. ) ;
#2211=DIRECTION ( 'NONE',  ( -1.357798298438996130E-15, 1.000000000000000000, 0.000000000000000000 ) ) ;
#2213=DIRECTION ( 'NONE',  ( 1.000000000000000000, 0.000000000000000000, 0.000000000000000000 ) ) ;
#2217=DIRECTION ( 'NONE',  ( 0.000000000000000000, 0.000000000000000000, -1.000000000000000000 ) ) ;
#2222=PLANE ( 'NONE',  #4879 ) ;
#2224=ORIENTED_EDGE ( 'NONE', *, *, #3717, .F. ) ;
#2226=CARTESIAN_POINT ( 'NONE',  ( 0.000000000000000000, 0.000000000000000000, -32.00000000000000000 ) ) ;
#2239=CARTESIAN_POINT ( 'NONE',  ( 15.00000000000000000, 20.00000000000000355, -20.00000000000000000 ) ) ;
#2240=VERTEX_POINT ( 'NONE', #943 ) ;
#2246=EDGE_LOOP ( 'NONE', ( #693, #3010, #1096, #4701, #563, #4382 ) ) ;
#2252=ADVANCED_FACE ( 'NONE', ( #3992 ), #1408, .T. ) ;
#2257=CARTESIAN_POINT ( 'NONE',  ( 25.00000000000000000, 16.00000000000000000, -26.00000000000000355 ) ) ;
#2262=AXIS2_PLACEMENT_3D ( 'NONE', #3150, #522, #1636 ) ;
#2269=CARTESIAN_POINT ( 'NONE',  ( 2.444036937190193033E-14, 6.999999999999999112, -32.00000000000000000 ) ) ;
#2277=DIRECTION ( 'NONE',  ( 0.000000000000000000, 0.000000000000000000, -1.000000000000000000 ) ) ;
#2280=ADVANCED_FACE ( 'NONE', ( #1322 ), #4414, .F. ) ;
#2281=CARTESIAN_POINT ( 'NONE',  ( 22.82279522939548144, 10.20431389251127463, -27.60486197633221650 ) ) ;
#2286=EDGE_CURVE ( 'NONE', #4866, #3891, #298, .T. ) ;
#2291=CARTESIAN_POINT ( 'NONE',  ( 22.35373982437574014, 11.19469724424307167, -32.00000000000000711 ) ) ;
#2294=DIRECTION ( 'NONE',  ( 0.000000000000000000, 0.000000000000000000, -1.000000000000000000 ) ) ;
#2314=CARTESIAN_POINT ( 'NONE',  ( 21.90226041726126383, -12.05376714070079025, -20.67955005196816032 ) ) ;
#2321=DIRECTION ( 'NONE',  ( -1.000000000000000000, -0.000000000000000000, -0.000000000000000000 ) ) ;
#2322=SURFACE_STYLE_FILL_AREA ( #787 ) ;
#2331=VECTOR ( 'NONE', #2950, 1000.000000000000000 ) ;
#2341=CARTESIAN_POINT ( 'NONE',  ( 6.999999999999999112, 0.000000000000000000, -32.00000000000000000 ) ) ;
#2344=AXIS2_PLACEMENT_3D ( 'NONE', #3895, #3550, #2430 ) ;
#2353=DIRECTION ( 'NONE',  ( -1.000000000000000000, 0.000000000000000000, 0.000000000000000000 ) ) ;
#2361=ORIENTED_EDGE ( 'NONE', *, *, #4579, .T. ) ;
#2363=CARTESIAN_POINT ( 'NONE',  ( 22.91733123609770928, -9.989778454058074075, -26.00578286613768597 ) ) ;
#2364=CARTESIAN_POINT ( 'NONE',  ( 15.00000000000000000, -11.10102051443364424, -20.00000000000000000 ) ) ;
#2366=VERTEX_POINT ( 'NONE', #3393 ) ;
#2373=ORIENTED_EDGE ( 'NONE', *, *, #3996, .F. ) ;
#2376=CARTESIAN_POINT ( 'NONE',  ( 15.00000000000000178, 16.00000000000000000, -28.64999999999998792 ) ) ;
#2377=EDGE_LOOP ( 'NONE', ( #114, #3510 ) ) ;
#2380=DIRECTION ( 'NONE',  ( -1.000000000000000000, 0.000000000000000000, 0.000000000000000000 ) ) ;
#2381=CARTESIAN_POINT ( 'NONE',  ( 0.000000000000000000, -11.10102051443364068, -32.00000000000000000 ) ) ;
#2382=ORIENTED_EDGE ( 'NONE', *, *, #4563, .F. ) ;
#2388=CARTESIAN_POINT ( 'NONE',  ( 15.00000000000000000, -16.00000000000000000, -26.00000000000000355 ) ) ;
#2390=ORIENTED_EDGE ( 'NONE', *, *, #1673, .F. ) ;
#2402=ORIENTED_EDGE ( 'NONE', *, *, #963, .T. ) ;
#2405=AXIS2_PLACEMENT_3D ( 'NONE', #4102, #618, #3726 ) ;
#2408=VECTOR ( 'NONE', #1867, 1000.000000000000000 ) ;
#2416=VERTEX_POINT ( 'NONE', #4510 ) ;
#2421=CYLINDRICAL_SURFACE ( 'NONE', #1700, 1.000000000000000888 ) ;
#2423=VECTOR ( 'NONE', #310, 1000.000000000000000 ) ;
#2424=ORIENTED_EDGE ( 'NONE', *, *, #870, .F. ) ;
#2429=CIRCLE ( 'NONE', #3066, 25.00000000000000000 ) ;
#2430=DIRECTION ( 'NONE',  ( 0.000000000000000000, 0.000000000000000000, -1.000000000000000000 ) ) ;
#2433=DIRECTION ( 'NONE',  ( -0.000000000000000000, -0.000000000000000000, 1.000000000000000000 ) ) ;
#2443=EDGE_LOOP ( 'NONE', ( #3923, #1646, #847, #3769 ) ) ;
#2456=VERTEX_POINT ( 'NONE', #4483 ) ;
#2462=DIRECTION ( 'NONE',  ( -1.000000000000000000, 0.000000000000000000, 0.000000000000000000 ) ) ;
#2464=CARTESIAN_POINT ( 'NONE',  ( 21.96462198364264395, -11.94070939570634948, -21.57727627927737046 ) ) ;
#2472=EDGE_CURVE ( 'NONE', #3165, #1024, #2495, .T. ) ;
#2475=DIRECTION ( 'NONE',  ( 1.000000000000000000, -0.000000000000000000, -0.000000000000000000 ) ) ;
#2477=CARTESIAN_POINT ( 'NONE',  ( 25.00000000000000000, 0.000000000000000000, -32.00000000000000000 ) ) ;
#2480=CARTESIAN_POINT ( 'NONE',  ( 0.000000000000000000, 0.000000000000000000, -32.00000000000000000 ) ) ;
#2487=CARTESIAN_POINT ( 'NONE',  ( 0.000000000000000000, 0.000000000000000000, -20.00000000000000000 ) ) ;
#2489=ORIENTED_EDGE ( 'NONE', *, *, #4160, .T. ) ;
#2494=DIRECTION ( 'NONE',  ( -1.000000000000000000, 0.000000000000000000, 0.000000000000000000 ) ) ;
#2495=CIRCLE ( 'NONE', #3448, 25.00000000000000000 ) ;
#2514=ORIENTED_EDGE ( 'NONE', *, *, #489, .F. ) ;
#2528=DIRECTION ( 'NONE',  ( -0.000000000000000000, -0.000000000000000000, 1.000000000000000000 ) ) ;
#2542=CARTESIAN_POINT ( 'NONE',  ( 22.30741055306794607, 11.28818263778244813, -19.99999999999996092 ) ) ;
#2544=ORIENTED_EDGE ( 'NONE', *, *, #4499, .T. ) ;
#2553=ORIENTED_EDGE ( 'NONE', *, *, #4499, .F. ) ;
#2554=CIRCLE ( 'NONE', #1829, 6.999999999999999112 ) ;
#2563=AXIS2_PLACEMENT_3D ( 'NONE', #2203, #3030, #2646 ) ;
#2566=CARTESIAN_POINT ( 'NONE',  ( 0.000000000000000000, 0.000000000000000000, -32.00000000000000000 ) ) ;
#2569=VERTEX_POINT ( 'NONE', #4666 ) ;
#2570=CARTESIAN_POINT ( 'NONE',  ( 15.00000000000000000, -16.00000000000000000, -26.00000000000000355 ) ) ;
#2571=FACE_OUTER_BOUND ( 'NONE', #3553, .T. ) ;
#2574=AXIS2_PLACEMENT_3D ( 'NONE', #3023, #730, #1811 ) ;
#2592=ADVANCED_FACE ( 'NONE', ( #862 ), #4313, .T. ) ;
#2596=DIRECTION ( 'NONE',  ( -1.000000000000000000, 0.000000000000000000, 0.000000000000000000 ) ) ;
#2597=VERTEX_POINT ( 'NONE', #2696 ) ;
#2623=DIRECTION ( 'NONE',  ( 1.000000000000000000, 0.000000000000000000, -0.000000000000000000 ) ) ;
#2627=EDGE_CURVE ( 'NONE', #987, #1875, #839, .T. ) ;
#2629=CARTESIAN_POINT ( 'NONE',  ( 15.00000000000000000, -16.00000000000000000, -23.35000000000000853 ) ) ;
#2631=CYLINDRICAL_SURFACE ( 'NONE', #4817, 5.999999999999998224 ) ;
#2637=AXIS2_PLACEMENT_3D ( 'NONE', #2226, #1769, #4834 ) ;
#2640=CARTESIAN_POINT ( 'NONE',  ( 22.21646894734066180, 11.46466559648295558, -31.93615172764430099 ) ) ;
#2645=DIRECTION ( 'NONE',  ( 0.000000000000000000, 0.000000000000000000, 1.000000000000000000 ) ) ;
#2646=DIRECTION ( 'NONE',  ( 0.000000000000000000, 0.000000000000000000, 1.000000000000000000 ) ) ;
#2648=( NAMED_UNIT ( * ) SI_UNIT ( $, .STERADIAN. ) SOLID_ANGLE_UNIT ( ) );
#2656=CIRCLE ( 'NONE', #3449, 2.649999999999985700 ) ;
#2658=ADVANCED_FACE ( 'NONE', ( #230 ), #2090, .F. ) ;
#2659=EDGE_CURVE ( 'NONE', #1875, #1889, #4088, .T. ) ;
#2660=CIRCLE ( 'NONE', #4412, 5.999999999999998224 ) ;
#2662=CARTESIAN_POINT ( 'NONE',  ( 22.47709430538512621, 10.94511065053865551, -29.23824484466006979 ) ) ;
#2664=DIRECTION ( 'NONE',  ( -0.000000000000000000, -0.000000000000000000, 1.000000000000000000 ) ) ;
#2667=APPLICATION_CONTEXT ( 'automotive_design' ) ;
#2672=FACE_OUTER_BOUND ( 'NONE', #4327, .T. ) ;
#2675=ORIENTED_EDGE ( 'NONE', *, *, #2110, .F. ) ;
#2676=VECTOR ( 'NONE', #3736, 1000.000000000000000 ) ;
#2678=DIRECTION ( 'NONE',  ( 1.000000000000000000, 0.000000000000000000, 0.000000000000000000 ) ) ;
#2682=CARTESIAN_POINT ( 'NONE',  ( -3.642919299551294898E-14, 16.00000000000000000, -23.35000000000000497 ) ) ;
#2687=CARTESIAN_POINT ( 'NONE',  ( 22.61871848390502393, 10.64917431867735154, -28.72182649103004692 ) ) ;
#2692=VERTEX_POINT ( 'NONE', #604 ) ;
#2693=CARTESIAN_POINT ( 'NONE',  ( -3.666055405785289392E-14, -6.999999999999999112, -20.00000000000000000 ) ) ;
#2696=CARTESIAN_POINT ( 'NONE',  ( 22.03949535914419755, -11.80087472665740478, -30.28571428571428470 ) ) ;
#2697=CARTESIAN_POINT ( 'NONE',  ( 21.96462198364264395, 11.94070939570634948, -30.42272372072263664 ) ) ;
#2700=DIRECTION ( 'NONE',  ( 0.000000000000000000, 0.000000000000000000, 1.000000000000000000 ) ) ;
#2705=UNCERTAINTY_MEASURE_WITH_UNIT (LENGTH_MEASURE( 1.000000000000000082E-05 ), #2021, 'distance_accuracy_value', 'NONE');
#2716=CARTESIAN_POINT ( 'NONE',  ( 0.000000000000000000, 0.000000000000000000, -32.00000000000000000 ) ) ;
#2719=EDGE_LOOP ( 'NONE', ( #4535, #160, #1611, #3257 ) ) ;
#2720=CIRCLE ( 'NONE', #2405, 6.999999999999999112 ) ;
#2731=ORIENTED_EDGE ( 'NONE', *, *, #628, .T. ) ;
#2736=CARTESIAN_POINT ( 'NONE',  ( 22.90825000241674303, -10.01062433489519954, -26.41097745015308718 ) ) ;
#2749=CARTESIAN_POINT ( 'NONE',  ( 21.87533763385574659, 12.10248395817102107, -30.91117611071771165 ) ) ;
#2755=B_SPLINE_CURVE_WITH_KNOTS ( 'NONE', 3,
 ( #4449, #4150, #1878, #4839, #1026, #4076, #2187, #284, #1805, #797, #464, #3823, #831, #3456, #25, #3858, #2281, #3485, #437, #2687, #3904, #2662, #1979, #1959, #3036 ),
 .UNSPECIFIED., .F., .F.,
 ( 4, 2, 2, 2, 2, 2, 1, 2, 2, 2, 2, 2, 4 ),
 ( 0.005424949174462414224, 0.006631086198200492922, 0.007234154710069537475, 0.007837223221938582896, 0.009043360245676663328, 0.009646428757545708749, 0.01024949726941475417, 0.01085256578128379785, 0.01145563429315284328, 0.01266177131689092197, 0.01326483982875995699, 0.01386790834062899200, 0.01507404536436706549 ),
 .UNSPECIFIED. ) ;
#2756=( NAMED_UNIT ( * ) PLANE_ANGLE_UNIT ( ) SI_UNIT ( $, .RADIAN. ) );
#2767=CARTESIAN_POINT ( 'NONE',  ( 22.47709430538511910, -10.94511065053865373, -22.76175515533994087 ) ) ;
#2775=CARTESIAN_POINT ( 'NONE',  ( 15.00000000000000000, -20.00000000000000355, -32.00000000000000000 ) ) ;
#2786=ORIENTED_EDGE ( 'NONE', *, *, #4081, .T. ) ;
#2787=ORIENTED_EDGE ( 'NONE', *, *, #1787, .T. ) ;
#2791=DIRECTION ( 'NONE',  ( -0.000000000000000000, -0.000000000000000000, 1.000000000000000000 ) ) ;
#2805=VECTOR ( 'NONE', #2838, 1000.000000000000000 ) ;
#2811=VERTEX_POINT ( 'NONE', #1081 ) ;
#2814=LINE ( 'NONE', #4658, #1307 ) ;
#2818=ORIENTED_EDGE ( 'NONE', *, *, #4660, .F. ) ;
#2819=ORIENTED_EDGE ( 'NONE', *, *, #2472, .T. ) ;
#2838=DIRECTION ( 'NONE',  ( -1.000000000000000000, 0.000000000000000000, 0.000000000000000000 ) ) ;
#2852=EDGE_CURVE ( 'NONE', #4670, #586, #1424, .T. ) ;
#2858=( NAMED_UNIT ( * ) SI_UNIT ( $, .STERADIAN. ) SOLID_ANGLE_UNIT ( ) );
#2865=EDGE_LOOP ( 'NONE', ( #2787, #2373, #864, #821 ) ) ;
#2874=ORIENTED_EDGE ( 'NONE', *, *, #1745, .F. ) ;
#2875=( GEOMETRIC_REPRESENTATION_CONTEXT ( 3 ) GLOBAL_UNCERTAINTY_ASSIGNED_CONTEXT ( ( #2705 ) ) GLOBAL_UNIT_ASSIGNED_CONTEXT ( ( #2021, #2756, #1219 ) ) REPRESENTATION_CONTEXT ( 'NONE', 'WORKASPACE' ) );
#2882=CARTESIAN_POINT ( 'NONE',  ( 15.00000000000000000, 16.00000000000000000, -28.64999999999999503 ) ) ;
#2885=FACE_OUTER_BOUND ( 'NONE', #4922, .T. ) ;
#2902=ORIENTED_EDGE ( 'NONE', *, *, #4579, .F. ) ;
#2907=ADVANCED_FACE ( 'NONE', ( #1475 ), #649, .F. ) ;
#2912=CIRCLE ( 'NONE', #3309, 25.00000000000000000 ) ;
#2924=DIRECTION ( 'NONE',  ( -0.000000000000000000, -0.000000000000000000, 1.000000000000000000 ) ) ;
#2928=CARTESIAN_POINT ( 'NONE',  ( 22.03949535914419755, -11.80087472665740478, -30.28571428571428470 ) ) ;
#2939=ORIENTED_EDGE ( 'NONE', *, *, #849, .T. ) ;
#2940=ORIENTED_EDGE ( 'NONE', *, *, #1703, .F. ) ;
#2942=CARTESIAN_POINT ( 'NONE',  ( 15.00000000000000000, -16.00000000000000000, -26.00000000000000355 ) ) ;
#2943=ORIENTED_EDGE ( 'NONE', *, *, #749, .T. ) ;
#2944=LINE ( 'NONE', #705, #191 ) ;
#2950=DIRECTION ( 'NONE',  ( 1.000000000000000000, -0.000000000000000000, -0.000000000000000000 ) ) ;
#2964=AXIS2_PLACEMENT_3D ( 'NONE', #3255, #1670, #965 ) ;
#2966=ORIENTED_EDGE ( 'NONE', *, *, #880, .T. ) ;
#2981=VECTOR ( 'NONE', #3801, 1000.000000000000000 ) ;
#2999=ORIENTED_EDGE ( 'NONE', *, *, #1396, .T. ) ;
#3002=LINE ( 'NONE', #3690, #2676 ) ;
#3010=ORIENTED_EDGE ( 'NONE', *, *, #3262, .T. ) ;
#3018=LINE ( 'NONE', #4527, #1143 ) ;
#3023=CARTESIAN_POINT ( 'NONE',  ( 0.000000000000000000, 0.000000000000000000, -20.00000000000000000 ) ) ;
#3025=CARTESIAN_POINT ( 'NONE',  ( 21.97815564317848924, -11.91494984865602902, -20.41093891521751047 ) ) ;
#3030=DIRECTION ( 'NONE',  ( -1.000000000000000000, -0.000000000000000000, 0.000000000000000000 ) ) ;
#3031=ADVANCED_FACE ( 'NONE', ( #3906, #4224 ), #3069, .F. ) ;
#3034=ORIENTED_EDGE ( 'NONE', *, *, #3675, .F. ) ;
#3036=CARTESIAN_POINT ( 'NONE',  ( 22.03949535914419755, 11.80087472665740300, -30.28571428571428470 ) ) ;
#3041=ORIENTED_EDGE ( 'NONE', *, *, #628, .F. ) ;
#3049=VECTOR ( 'NONE', #4044, 1000.000000000000000 ) ;
#3062=AXIS2_PLACEMENT_3D ( 'NONE', #155, #1728, #4340 ) ;
#3063=CIRCLE ( 'NONE', #6, 25.00000000000000000 ) ;
#3066=AXIS2_PLACEMENT_3D ( 'NONE', #935, #916, #2462 ) ;
#3067=CARTESIAN_POINT ( 'NONE',  ( 22.88998946896871800, -10.05230818559221717, -26.81638557257617705 ) ) ;
#3069=PLANE ( 'NONE',  #4249 ) ;
#3072=AXIS2_PLACEMENT_3D ( 'NONE', #1714, #4846, #4389 ) ;
#3089=DIRECTION ( 'NONE',  ( 1.000000000000000000, -0.000000000000000000, -0.000000000000000000 ) ) ;
#3091=ORIENTED_EDGE ( 'NONE', *, *, #2627, .T. ) ;
#3099=DIRECTION ( 'NONE',  ( 0.000000000000000000, 0.000000000000000000, -1.000000000000000000 ) ) ;
#3103=ORIENTED_EDGE ( 'NONE', *, *, #3540, .T. ) ;
#3105=DIRECTION ( 'NONE',  ( -1.000000000000000000, 0.000000000000000000, 0.000000000000000000 ) ) ;
#3112=ORIENTED_EDGE ( 'NONE', *, *, #1060, .F. ) ;
#3118=ORIENTED_EDGE ( 'NONE', *, *, #966, .T. ) ;
#3123=CARTESIAN_POINT ( 'NONE',  ( 22.40016391766193493, 11.10102051443364068, -32.00000000000000000 ) ) ;
#3126=VERTEX_POINT ( 'NONE', #3628 ) ;
#3138=CARTESIAN_POINT ( 'NONE',  ( 22.89074894326664378, -10.05057747304974569, -25.19644245487525325 ) ) ;
#3143=ORIENTED_EDGE ( 'NONE', *, *, #4830, .T. ) ;
#3150=CARTESIAN_POINT ( 'NONE',  ( -3.642919299551294898E-14, -16.00000000000000000, -26.00000000000000355 ) ) ;
#3152=EDGE_CURVE ( 'NONE', #1695, #4670, #1303, .T. ) ;
#3162=FACE_OUTER_BOUND ( 'NONE', #1225, .T. ) ;
#3165=VERTEX_POINT ( 'NONE', #992 ) ;
#3174=CARTESIAN_POINT ( 'NONE',  ( 0.000000000000000000, 0.000000000000000000, -32.00000000000000000 ) ) ;
#3183=ORIENTED_EDGE ( 'NONE', *, *, #2852, .T. ) ;
#3185=LINE ( 'NONE', #4726, #4470 ) ;
#3191=ORIENTED_EDGE ( 'NONE', *, *, #2204, .F. ) ;
#3192=CARTESIAN_POINT ( 'NONE',  ( 0.000000000000000000, 0.000000000000000000, -20.00000000000000000 ) ) ;
#3195=ORIENTED_EDGE ( 'NONE', *, *, #684, .F. ) ;
#3196=EDGE_CURVE ( 'NONE', #4670, #1695, #651, .T. ) ;
#3199=PRODUCT_DEFINITION_FORMATION_WITH_SPECIFIED_SOURCE ( 'ANY', '', #263, .NOT_KNOWN. ) ;
#3206=CYLINDRICAL_SURFACE ( 'NONE', #2964, 25.00000000000000000 ) ;
#3207=LINE ( 'NONE', #2381, #4155 ) ;
#3217=VERTEX_POINT ( 'NONE', #1069 ) ;
#3218=ORIENTED_EDGE ( 'NONE', *, *, #1745, .T. ) ;
#3219=AXIS2_PLACEMENT_3D ( 'NONE', #1756, #2494, #588 ) ;
#3229=CARTESIAN_POINT ( 'NONE',  ( 21.90877321452243010, 12.04191644460182609, -21.39663540706808575 ) ) ;
#3232=VECTOR ( 'NONE', #1598, 1000.000000000000000 ) ;
#3239=PLANE ( 'NONE',  #4111 ) ;
#3246=CARTESIAN_POINT ( 'NONE',  ( -3.642919299551294898E-14, 16.00000000000000000, -28.64999999999999858 ) ) ;
#3247=EDGE_CURVE ( 'NONE', #4690, #2692, #2660, .T. ) ;
#3255=CARTESIAN_POINT ( 'NONE',  ( 0.000000000000000000, 0.000000000000000000, -32.00000000000000000 ) ) ;
#3257=ORIENTED_EDGE ( 'NONE', *, *, #1544, .T. ) ;
#3261=VERTEX_POINT ( 'NONE', #4901 ) ;
#3262=EDGE_CURVE ( 'NONE', #3494, #4690, #4740, .T. ) ;
#3265=FACE_OUTER_BOUND ( 'NONE', #1163, .T. ) ;
#3274=EDGE_LOOP ( 'NONE', ( #4910, #2818, #3103, #2075 ) ) ;
#3276=CARTESIAN_POINT ( 'NONE',  ( 22.40016391766193493, -11.10102051443364068, -32.00000000000000000 ) ) ;
#3287=ORIENTED_EDGE ( 'NONE', *, *, #1673, .T. ) ;
#3292=CARTESIAN_POINT ( 'NONE',  ( 21.96482728828171460, 11.94032596560094817, -21.57765196252147177 ) ) ;
#3298=ORIENTED_EDGE ( 'NONE', *, *, #2659, .F. ) ;
#3302=FACE_OUTER_BOUND ( 'NONE', #4865, .T. ) ;
#3306=AXIS2_PLACEMENT_3D ( 'NONE', #2190, #260, #307 ) ;
#3309=AXIS2_PLACEMENT_3D ( 'NONE', #696, #3746, #2353 ) ;
#3317=ORIENTED_EDGE ( 'NONE', *, *, #2204, .T. ) ;
#3335=FACE_OUTER_BOUND ( 'NONE', #3820, .T. ) ;
#3343=EDGE_CURVE ( 'NONE', #1024, #3700, #688, .T. ) ;
#3346=CARTESIAN_POINT ( 'NONE',  ( 25.00000000000000000, -16.00000000000000000, -26.00000000000000355 ) ) ;
#3349=ADVANCED_FACE ( 'NONE', ( #636, #1145 ), #1835, .F. ) ;
#3359=CARTESIAN_POINT ( 'NONE',  ( 0.000000000000000000, 0.000000000000000000, -32.00000000000000000 ) ) ;
#3367=ORIENTED_EDGE ( 'NONE', *, *, #3152, .F. ) ;
#3368=CARTESIAN_POINT ( 'NONE',  ( 0.000000000000000000, -25.00000000000000000, -32.00000000000000000 ) ) ;
#3369=CARTESIAN_POINT ( 'NONE',  ( 15.00000000000000000, 16.00000000000000000, -26.00000000000000355 ) ) ;
#3372=AXIS2_PLACEMENT_3D ( 'NONE', #4558, #364, #1886 ) ;
#3378=ADVANCED_FACE ( 'NONE', ( #699, #3386 ), #376, .F. ) ;
#3385=LINE ( 'NONE', #4939, #2181 ) ;
#3386=FACE_OUTER_BOUND ( 'NONE', #4498, .T. ) ;
#3393=CARTESIAN_POINT ( 'NONE',  ( 0.000000000000000000, -25.00000000000000000, -20.00000000000000000 ) ) ;
#3399=CARTESIAN_POINT ( 'NONE',  ( 25.00000000000000000, 11.80087472665741011, -21.71428571428571530 ) ) ;
#3406=CARTESIAN_POINT ( 'NONE',  ( 6.999999999999999112, 0.000000000000000000, -20.00000000000000000 ) ) ;
#3415=CARTESIAN_POINT ( 'NONE',  ( 22.03949535914419755, 11.80087472665740300, -30.28571428571428470 ) ) ;
#3429=CARTESIAN_POINT ( 'NONE',  ( 22.65824501284922476, -10.56463292904779827, -28.54887252943416343 ) ) ;
#3439=CARTESIAN_POINT ( 'NONE',  ( 21.90822715901080642, 12.04290832652441168, -30.60487698215225194 ) ) ;
#3448=AXIS2_PLACEMENT_3D ( 'NONE', #2566, #1812, #2596 ) ;
#3449=AXIS2_PLACEMENT_3D ( 'NONE', #4457, #3759, #2217 ) ;
#3450=CARTESIAN_POINT ( 'NONE',  ( 15.00000000000000000, -11.80087472665740300, -30.28571428571428470 ) ) ;
#3456=CARTESIAN_POINT ( 'NONE',  ( 22.90859662698202825, 10.00982993400316978, -26.39899337456353123 ) ) ;
#3461=ORIENTED_EDGE ( 'NONE', *, *, #4081, .F. ) ;
#3485=CARTESIAN_POINT ( 'NONE',  ( 22.76902711785762889, 10.32479573876449130, -27.98806281106213589 ) ) ;
#3488=ORIENTED_EDGE ( 'NONE', *, *, #749, .F. ) ;
#3494=VERTEX_POINT ( 'NONE', #878 ) ;
#3499=ORIENTED_EDGE ( 'NONE', *, *, #1951, .T. ) ;
#3504=CARTESIAN_POINT ( 'NONE',  ( 22.52496067886514552, -10.84608396733234237, -29.07843770730522337 ) ) ;
#3510=ORIENTED_EDGE ( 'NONE', *, *, #4141, .T. ) ;
#3514=CARTESIAN_POINT ( 'NONE',  ( 21.90822715901080642, -12.04290832652441168, -21.39512301784776227 ) ) ;
#3520=CARTESIAN_POINT ( 'NONE',  ( 15.00000000000000000, -16.00000000000000000, -20.00000000000000000 ) ) ;
#3524=AXIS2_PLACEMENT_3D ( 'NONE', #395, #1921, #2277 ) ;
#3525=EDGE_LOOP ( 'NONE', ( #2940, #3091, #827, #1957 ) ) ;
#3531=VECTOR ( 'NONE', #1965, 1000.000000000000000 ) ;
#3532=CARTESIAN_POINT ( 'NONE',  ( 22.18564505841182211, -11.52792329777113878, -21.98172240441969905 ) ) ;
#3540=EDGE_CURVE ( 'NONE', #3700, #165, #2814, .T. ) ;
#3548=ORIENTED_EDGE ( 'NONE', *, *, #684, .T. ) ;
#3550=DIRECTION ( 'NONE',  ( 1.000000000000000000, -0.000000000000000000, -0.000000000000000000 ) ) ;
#3553=EDGE_LOOP ( 'NONE', ( #23, #2361, #1656, #2402, #3562, #180 ) ) ;
#3562=ORIENTED_EDGE ( 'NONE', *, *, #1060, .T. ) ;
#3575=FACE_OUTER_BOUND ( 'NONE', #4112, .T. ) ;
#3590=CARTESIAN_POINT ( 'NONE',  ( 22.04417985544612790, 11.79351823160730461, -20.25405616187230962 ) ) ;
#3592=ORIENTED_EDGE ( 'NONE', *, *, #1917, .F. ) ;
#3596=ORIENTED_EDGE ( 'NONE', *, *, #1515, .F. ) ;
#3599=EDGE_CURVE ( 'NONE', #3261, #1067, #932, .T. ) ;
#3600=DIRECTION ( 'NONE',  ( 0.000000000000000000, 0.000000000000000000, 1.000000000000000000 ) ) ;
#3602=ORIENTED_EDGE ( 'NONE', *, *, #4116, .F. ) ;
#3603=VERTEX_POINT ( 'NONE', #2364 ) ;
#3613=AXIS2_PLACEMENT_3D ( 'NONE', #4514, #4140, #710 ) ;
#3624=EDGE_LOOP ( 'NONE', ( #3838, #1972 ) ) ;
#3628=CARTESIAN_POINT ( 'NONE',  ( 15.00000000000000000, 11.80087472665740300, -30.28571428571428470 ) ) ;
#3633=DIRECTION ( 'NONE',  ( -1.000000000000000000, 0.000000000000000000, 0.000000000000000000 ) ) ;
#3647=PRODUCT_CONTEXT ( 'NONE', #3945, 'mechanical' ) ;
#3650=CARTESIAN_POINT ( 'NONE',  ( -3.642919299551294898E-14, 16.00000000000000000, -26.00000000000000355 ) ) ;
#3656=CYLINDRICAL_SURFACE ( 'NONE', #101, 25.00000000000000000 ) ;
#3657=VERTEX_POINT ( 'NONE', #2376 ) ;
#3661=CARTESIAN_POINT ( 'NONE',  ( 21.86452818504794138, 12.12206676558875529, -20.99167230228674441 ) ) ;
#3668=DIRECTION ( 'NONE',  ( -0.000000000000000000, -1.000000000000000000, -0.000000000000000000 ) ) ;
#3675=EDGE_CURVE ( 'NONE', #3891, #2240, #2912, .T. ) ;
#3690=CARTESIAN_POINT ( 'NONE',  ( 2.444036937190193033E-14, 6.999999999999999112, -32.00000000000000000 ) ) ;
#3700=VERTEX_POINT ( 'NONE', #4497 ) ;
#3707=CARTESIAN_POINT ( 'NONE',  ( 15.00000000000000000, 16.00000000000000000, -23.35000000000000853 ) ) ;
#3713=EDGE_CURVE ( 'NONE', #3603, #2165, #1224, .T. ) ;
#3717=EDGE_CURVE ( 'NONE', #4613, #1731, #4258, .T. ) ;
#3726=DIRECTION ( 'NONE',  ( -1.000000000000000000, 0.000000000000000000, 0.000000000000000000 ) ) ;
#3736=DIRECTION ( 'NONE',  ( -0.000000000000000000, -0.000000000000000000, 1.000000000000000000 ) ) ;
#3746=DIRECTION ( 'NONE',  ( 0.000000000000000000, 0.000000000000000000, -1.000000000000000000 ) ) ;
#3757=ORIENTED_EDGE ( 'NONE', *, *, #1366, .F. ) ;
#3759=DIRECTION ( 'NONE',  ( 1.000000000000000000, -0.000000000000000000, -0.000000000000000000 ) ) ;
#3766=CARTESIAN_POINT ( 'NONE',  ( 15.00000000000000000, 11.10102051443364424, -20.00000000000000000 ) ) ;
#3769=ORIENTED_EDGE ( 'NONE', *, *, #113, .F. ) ;
#3774=AXIS2_PLACEMENT_3D ( 'NONE', #2269, #4096, #1816 ) ;
#3776=STYLED_ITEM ( 'NONE', ( #620 ), #2079 ) ;
#3801=DIRECTION ( 'NONE',  ( 1.000000000000000000, -0.000000000000000000, -0.000000000000000000 ) ) ;
#3807=DIRECTION ( 'NONE',  ( -1.000000000000000000, 0.000000000000000000, 0.000000000000000000 ) ) ;
#3809=CARTESIAN_POINT ( 'NONE',  ( 22.04753367391287000, 11.78607713658132639, -31.73496350056613480 ) ) ;
#3820=EDGE_LOOP ( 'NONE', ( #4368, #2939, #512, #1036 ) ) ;
#3823=CARTESIAN_POINT ( 'NONE',  ( 22.90825000241675014, 10.01062433489520132, -25.58902254984691638 ) ) ;
#3833=CYLINDRICAL_SURFACE ( 'NONE', #2100, 6.999999999999999112 ) ;
#3835=CARTESIAN_POINT ( 'NONE',  ( 22.08746549892786604, 11.71119031839157820, -31.79783224586644508 ) ) ;
#3838=ORIENTED_EDGE ( 'NONE', *, *, #1544, .F. ) ;
#3856=VECTOR ( 'NONE', #4365, 1000.000000000000000 ) ;
#3858=CARTESIAN_POINT ( 'NONE',  ( 22.87713223651540417, 10.08160808888849047, -27.00698909695861261 ) ) ;
#3874=FACE_OUTER_BOUND ( 'NONE', #1258, .T. ) ;
#3891=VERTEX_POINT ( 'NONE', #4721 ) ;
#3895=CARTESIAN_POINT ( 'NONE',  ( 15.00000000000000000, 16.00000000000000000, -26.00000000000000355 ) ) ;
#3901=EDGE_LOOP ( 'NONE', ( #3195, #1899, #1988, #3041 ) ) ;
#3902=EDGE_CURVE ( 'NONE', #3261, #1889, #3002, .T. ) ;
#3904=CARTESIAN_POINT ( 'NONE',  ( 22.52717933085840585, 10.84147272832753828, -29.07071185665252600 ) ) ;
#3906=FACE_BOUND ( 'NONE', #3624, .T. ) ;
#3912=FACE_OUTER_BOUND ( 'NONE', #3525, .T. ) ;
#3923=ORIENTED_EDGE ( 'NONE', *, *, #4141, .F. ) ;
#3928=ORIENTED_EDGE ( 'NONE', *, *, #4446, .F. ) ;
#3929=EDGE_LOOP ( 'NONE', ( #4638, #3367, #2943, #1276 ) ) ;
#3932=CARTESIAN_POINT ( 'NONE',  ( 15.00000000000000000, -16.00000000000000000, -28.64999999999999503 ) ) ;
#3945=APPLICATION_CONTEXT ( 'automotive_design' ) ;
#3946=ORIENTED_EDGE ( 'NONE', *, *, #3599, .T. ) ;
#3954=DIRECTION ( 'NONE',  ( 1.000000000000000000, 0.000000000000000000, 0.000000000000000000 ) ) ;
#3968=ORIENTED_EDGE ( 'NONE', *, *, #3713, .F. ) ;
#3978=CARTESIAN_POINT ( 'NONE',  ( 2.444036937190193033E-14, 6.999999999999999112, -32.00000000000000000 ) ) ;
#3980=B_SPLINE_CURVE_WITH_KNOTS ( 'NONE', 3,
 ( #1534, #4265, #4594, #1192, #4208, #4233, #781, #3025, #1987, #2314, #807, #840, #472, #3514, #2464, #156 ),
 .UNSPECIFIED., .F., .F.,
 ( 4, 2, 2, 2, 2, 2, 2, 4 ),
 ( 0.000000000000000000, 0.0003092645584586379615, 0.0006185291169172759231, 0.0009277936753759138304, 0.001237058233834551846, 0.001546322792293189754, 0.001855587350751827661, 0.002474116467669114534 ),
 .UNSPECIFIED. ) ;
#3987=LINE ( 'NONE', #2775, #3856 ) ;
#3992=FACE_OUTER_BOUND ( 'NONE', #3901, .T. ) ;
#3994=VECTOR ( 'NONE', #3668, 1000.000000000000000 ) ;
#3995=LINE ( 'NONE', #145, #2805 ) ;
#3996=EDGE_CURVE ( 'NONE', #1067, #2416, #2944, .T. ) ;
#3997=LINE ( 'NONE', #2882, #3049 ) ;
#4000=VECTOR ( 'NONE', #2528, 1000.000000000000000 ) ;
#4001=DIRECTION ( 'NONE',  ( 0.000000000000000000, 0.000000000000000000, -1.000000000000000000 ) ) ;
#4003=VERTEX_POINT ( 'NONE', #2239 ) ;
#4009=AXIS2_PLACEMENT_3D ( 'NONE', #3192, #884, #1286 ) ;
#4019=ORIENTED_EDGE ( 'NONE', *, *, #3996, .T. ) ;
#4034=CARTESIAN_POINT ( 'NONE',  ( 22.40016391766193138, -11.10102051443364424, -20.00000000000000000 ) ) ;
#4043=FACE_BOUND ( 'NONE', #4773, .T. ) ;
#4044=DIRECTION ( 'NONE',  ( 1.000000000000000000, -0.000000000000000000, -0.000000000000000000 ) ) ;
#4050=SURFACE_STYLE_USAGE ( .BOTH. , #1743 ) ;
#4059=ORIENTED_EDGE ( 'NONE', *, *, #1478, .F. ) ;
#4061=CARTESIAN_POINT ( 'NONE',  ( 22.21307774062918128, 11.47223234890555688, -20.05227268063044832 ) ) ;
#4065=LINE ( 'NONE', #2129, #796 ) ;
#4067=VECTOR ( 'NONE', #4494, 1000.000000000000000 ) ;
#4076=CARTESIAN_POINT ( 'NONE',  ( 22.61674500023158885, 10.65336738338371880, -23.26995442300275130 ) ) ;
#4081=EDGE_CURVE ( 'NONE', #2811, #4838, #159, .T. ) ;
#4088=CIRCLE ( 'NONE', #4484, 6.999999999999999112 ) ;
#4091=ORIENTED_EDGE ( 'NONE', *, *, #4886, .T. ) ;
#4092=ORIENTED_EDGE ( 'NONE', *, *, #4830, .F. ) ;
#4096=DIRECTION ( 'NONE',  ( 1.000000000000000000, 1.357798298438996130E-15, 0.000000000000000000 ) ) ;
#4102=CARTESIAN_POINT ( 'NONE',  ( 0.000000000000000000, 0.000000000000000000, -20.00000000000000000 ) ) ;
#4111=AXIS2_PLACEMENT_3D ( 'NONE', #2480, #4001, #4397 ) ;
#4112=EDGE_LOOP ( 'NONE', ( #1828, #2489, #3218, #2553 ) ) ;
#4116=EDGE_CURVE ( 'NONE', #4310, #3217, #3980, .T. ) ;
#4126=ORIENTED_EDGE ( 'NONE', *, *, #880, .F. ) ;
#4127=DIRECTION ( 'NONE',  ( 0.000000000000000000, 0.000000000000000000, 1.000000000000000000 ) ) ;
#4140=DIRECTION ( 'NONE',  ( -1.000000000000000000, -0.000000000000000000, 0.000000000000000000 ) ) ;
#4141=EDGE_CURVE ( 'NONE', #2569, #181, #4570, .T. ) ;
#4150=CARTESIAN_POINT ( 'NONE',  ( 22.18526740102421257, 11.52862861652371507, -21.98103133599976289 ) ) ;
#4155=VECTOR ( 'NONE', #4727, 1000.000000000000000 ) ;
#4160=EDGE_CURVE ( 'NONE', #3165, #2165, #3987, .T. ) ;
#4180=DIRECTION ( 'NONE',  ( -0.000000000000000000, 1.000000000000000000, -0.000000000000000000 ) ) ;
#4183=LINE ( 'NONE', #3932, #4837 ) ;
#4187=CARTESIAN_POINT ( 'NONE',  ( 22.17126811103361206, 11.55175229948174120, -31.89759920908706547 ) ) ;
#4208=CARTESIAN_POINT ( 'NONE',  ( 22.17126811103361206, -11.55175229948174476, -20.10240079091293808 ) ) ;
#4218=VERTEX_POINT ( 'NONE', #1608 ) ;
#4221=SHAPE_REPRESENTATION ( 'locker', ( #1918 ), #1581 ) ;
#4222=CARTESIAN_POINT ( 'NONE',  ( 22.82142399877221450, -10.20738559227135944, -27.61557768215598685 ) ) ;
#4224=FACE_OUTER_BOUND ( 'NONE', #2246, .T. ) ;
#4233=CARTESIAN_POINT ( 'NONE',  ( 22.08746549892785893, -11.71119031839158176, -20.20216775413354426 ) ) ;
#4234=ADVANCED_FACE ( 'NONE', ( #4315 ), #2421, .T. ) ;
#4249=AXIS2_PLACEMENT_3D ( 'NONE', #2388, #4282, #833 ) ;
#4250=CIRCLE ( 'NONE', #4009, 25.00000000000000000 ) ;
#4254=CIRCLE ( 'NONE', #184, 25.00000000000000000 ) ;
#4258=CIRCLE ( 'NONE', #1230, 1.000000000000000888 ) ;
#4265=CARTESIAN_POINT ( 'NONE',  ( 22.35373982437574014, -11.19469724424307344, -20.00000000000000355 ) ) ;
#4267=CLOSED_SHELL ( 'NONE', ( #2093, #719, #1508, #4512, #4339, #4731, #1445, #4812, #3378, #2907, #3349, #381, #4920, #3031, #1846, #4919, #2592, #2252, #295, #4234, #2280, #2658 ) ) ;
#4270=CARTESIAN_POINT ( 'NONE',  ( 0.000000000000000000, 0.000000000000000000, -20.00000000000000000 ) ) ;
#4282=DIRECTION ( 'NONE',  ( -1.000000000000000000, -0.000000000000000000, 0.000000000000000000 ) ) ;
#4302=ORIENTED_EDGE ( 'NONE', *, *, #3540, .F. ) ;
#4303=EDGE_CURVE ( 'NONE', #3657, #586, #427, .T. ) ;
#4304=COLOUR_RGB ( '', 0.72549020, 0.75294118, 0.79215686) ;
#4310=VERTEX_POINT ( 'NONE', #4034 ) ;
#4313=CYLINDRICAL_SURFACE ( 'NONE', #21, 1.000000000000000888 ) ;
#4315=FACE_OUTER_BOUND ( 'NONE', #1539, .T. ) ;
#4327=EDGE_LOOP ( 'NONE', ( #3968, #3143, #2390, #3034, #2966, #2902, #2675, #371, #3298, #2382, #4917, #2874 ) ) ;
#4329=VECTOR ( 'NONE', #4665, 1000.000000000000000 ) ;
#4335=ORIENTED_EDGE ( 'NONE', *, *, #1478, .T. ) ;
#4337=( GEOMETRIC_REPRESENTATION_CONTEXT ( 3 ) GLOBAL_UNCERTAINTY_ASSIGNED_CONTEXT ( ( #1490 ) ) GLOBAL_UNIT_ASSIGNED_CONTEXT ( ( #4932, #347, #2648 ) ) REPRESENTATION_CONTEXT ( 'NONE', 'WORKASPACE' ) );
#4339=ADVANCED_FACE ( 'NONE', ( #3265 ), #3656, .T. ) ;
#4340=DIRECTION ( 'NONE',  ( 0.000000000000000000, 0.000000000000000000, -1.000000000000000000 ) ) ;
#4357=CARTESIAN_POINT ( 'NONE',  ( -3.642919299551294898E-14, -16.00000000000000000, -28.64999999999999858 ) ) ;
#4359=VERTEX_POINT ( 'NONE', #4452 ) ;
#4365=DIRECTION ( 'NONE',  ( -0.000000000000000000, -0.000000000000000000, 1.000000000000000000 ) ) ;
#4368=ORIENTED_EDGE ( 'NONE', *, *, #963, .F. ) ;
#4375=CARTESIAN_POINT ( 'NONE',  ( 21.87894646962818612, -12.09631101282777266, -31.22510989603295428 ) ) ;
#4382=ORIENTED_EDGE ( 'NONE', *, *, #4160, .F. ) ;
#4389=DIRECTION ( 'NONE',  ( -1.000000000000000000, 0.000000000000000000, 0.000000000000000000 ) ) ;
#4394=CARTESIAN_POINT ( 'NONE',  ( 21.86452818504794138, -12.12206676558875529, -31.00832769771325559 ) ) ;
#4397=DIRECTION ( 'NONE',  ( -1.000000000000000000, 0.000000000000000000, -0.000000000000000000 ) ) ;
#4403=DIRECTION ( 'NONE',  ( -0.000000000000000000, -0.000000000000000000, 1.000000000000000000 ) ) ;
#4412=AXIS2_PLACEMENT_3D ( 'NONE', #2570, #2623, #2645 ) ;
#4414=CYLINDRICAL_SURFACE ( 'NONE', #892, 2.649999999999992806 ) ;
#4440=CARTESIAN_POINT ( 'NONE',  ( 22.03949535914419400, 11.80087472665740655, -21.71428571428571885 ) ) ;
#4446=EDGE_CURVE ( 'NONE', #3165, #3494, #3018, .T. ) ;
#4449=CARTESIAN_POINT ( 'NONE',  ( 22.03949535914419400, 11.80087472665740655, -21.71428571428571885 ) ) ;
#4452=CARTESIAN_POINT ( 'NONE',  ( 15.00000000000000000, 11.10102051443364068, -32.00000000000000000 ) ) ;
#4457=CARTESIAN_POINT ( 'NONE',  ( 15.00000000000000178, 16.00000000000000000, -26.00000000000000355 ) ) ;
#4458=CARTESIAN_POINT ( 'NONE',  ( 21.97031423931356287, 11.92955703141275237, -20.40434499790757172 ) ) ;
#4467=AXIS2_PLACEMENT_3D ( 'NONE', #4755, #2433, #3954 ) ;
#4470=VECTOR ( 'NONE', #1413, 1000.000000000000000 ) ;
#4473=VECTOR ( 'NONE', #1624, 1000.000000000000000 ) ;
#4475=DIRECTION ( 'NONE',  ( -1.000000000000000000, 0.000000000000000000, 0.000000000000000000 ) ) ;
#4483=CARTESIAN_POINT ( 'NONE',  ( 15.00000000000000178, -16.00000000000000000, -28.64999999999998792 ) ) ;
#4484=AXIS2_PLACEMENT_3D ( 'NONE', #2487, #2119, #3633 ) ;
#4490=CARTESIAN_POINT ( 'NONE',  ( 22.03949535914419755, 11.80087472665740300, -30.28571428571428470 ) ) ;
#4494=DIRECTION ( 'NONE',  ( -0.000000000000000000, -0.000000000000000000, 1.000000000000000000 ) ) ;
#4497=CARTESIAN_POINT ( 'NONE',  ( -3.666055405785289392E-14, -6.999999999999999112, -32.00000000000000000 ) ) ;
#4498=EDGE_LOOP ( 'NONE', ( #1247, #4302, #2210, #2544 ) ) ;
#4499=EDGE_CURVE ( 'NONE', #1024, #2366, #1370, .T. ) ;
#4506=AXIS2_PLACEMENT_3D ( 'NONE', #221, #599, #3600 ) ;
#4510=CARTESIAN_POINT ( 'NONE',  ( 0.000000000000000000, 25.00000000000000000, -20.00000000000000000 ) ) ;
#4512=ADVANCED_FACE ( 'NONE', ( #2207 ), #1801, .T. ) ;
#4514=CARTESIAN_POINT ( 'NONE',  ( 15.00000000000000000, -11.10102051443364068, -31.00000000000000000 ) ) ;
#4515=DIRECTION ( 'NONE',  ( -1.000000000000000000, 0.000000000000000000, 0.000000000000000000 ) ) ;
#4527=CARTESIAN_POINT ( 'NONE',  ( 15.00000000000000000, -16.00000000000000000, -32.00000000000000000 ) ) ;
#4531=LINE ( 'NONE', #4948, #2423 ) ;
#4535=ORIENTED_EDGE ( 'NONE', *, *, #400, .F. ) ;
#4558=CARTESIAN_POINT ( 'NONE',  ( 0.000000000000000000, 0.000000000000000000, -32.00000000000000000 ) ) ;
#4561=VECTOR ( 'NONE', #2123, 1000.000000000000000 ) ;
#4563=EDGE_CURVE ( 'NONE', #165, #1875, #2720, .T. ) ;
#4570=CIRCLE ( 'NONE', #2262, 2.649999999999995914 ) ;
#4579=EDGE_CURVE ( 'NONE', #4003, #4613, #1843, .T. ) ;
#4583=CARTESIAN_POINT ( 'NONE',  ( 22.82279522939548144, -10.20431389251127285, -24.39513802366778705 ) ) ;
#4589=AXIS2_PLACEMENT_3D ( 'NONE', #4706, #1628, #1652 ) ;
#4593=DIRECTION ( 'NONE',  ( -1.000000000000000000, 0.000000000000000000, 0.000000000000000000 ) ) ;
#4594=CARTESIAN_POINT ( 'NONE',  ( 22.30769810302473033, -11.28612666381333440, -20.01290653110665119 ) ) ;
#4598=CARTESIAN_POINT ( 'NONE',  ( 0.000000000000000000, -25.00000000000000000, -32.00000000000000000 ) ) ;
#4613=VERTEX_POINT ( 'NONE', #394 ) ;
#4617=CARTESIAN_POINT ( 'NONE',  ( 21.88691174701116537, 12.08152700620044939, -31.22242340959439133 ) ) ;
#4625=DIRECTION ( 'NONE',  ( -0.000000000000000000, -0.000000000000000000, 1.000000000000000000 ) ) ;
#4636=DIRECTION ( 'NONE',  ( -0.000000000000000000, -0.000000000000000000, 1.000000000000000000 ) ) ;
#4638=ORIENTED_EDGE ( 'NONE', *, *, #2852, .F. ) ;
#4646=AXIS2_PLACEMENT_3D ( 'NONE', #1147, #2678, #2294 ) ;
#4657=CARTESIAN_POINT ( 'NONE',  ( 22.87713223651540417, -10.08160808888848514, -24.99301090304139095 ) ) ;
#4658=CARTESIAN_POINT ( 'NONE',  ( -3.666055405785289392E-14, -6.999999999999999112, -32.00000000000000000 ) ) ;
#4660=EDGE_CURVE ( 'NONE', #3700, #987, #2554, .T. ) ;
#4665=DIRECTION ( 'NONE',  ( -0.000000000000000000, -0.000000000000000000, 1.000000000000000000 ) ) ;
#4666=CARTESIAN_POINT ( 'NONE',  ( -3.642919299551294898E-14, -16.00000000000000000, -23.35000000000000497 ) ) ;
#4670=VERTEX_POINT ( 'NONE', #2682 ) ;
#4673=DIRECTION ( 'NONE',  ( 0.000000000000000000, 0.000000000000000000, -1.000000000000000000 ) ) ;
#4687=DIRECTION ( 'NONE',  ( 0.000000000000000000, 0.000000000000000000, -1.000000000000000000 ) ) ;
#4690=VERTEX_POINT ( 'NONE', #3450 ) ;
#4701=ORIENTED_EDGE ( 'NONE', *, *, #870, .T. ) ;
#4706=CARTESIAN_POINT ( 'NONE',  ( 15.00000000000000178, -16.00000000000000000, -26.00000000000000355 ) ) ;
#4712=CARTESIAN_POINT ( 'NONE',  ( 15.00000000000000000, 11.80087472665740655, -21.71428571428571885 ) ) ;
#4718=ORIENTED_EDGE ( 'NONE', *, *, #4737, .F. ) ;
#4721=CARTESIAN_POINT ( 'NONE',  ( 22.40016391766193138, 11.10102051443364424, -20.00000000000000000 ) ) ;
#4723=CIRCLE ( 'NONE', #2563, 1.000000000000000888 ) ;
#4726=CARTESIAN_POINT ( 'NONE',  ( 19.20937271229854915, -11.10102051443364424, -20.00000000000000000 ) ) ;
#4727=DIRECTION ( 'NONE',  ( -1.000000000000000000, 0.000000000000000000, 0.000000000000000000 ) ) ;
#4728=VECTOR ( 'NONE', #1434, 1000.000000000000000 ) ;
#4731=ADVANCED_FACE ( 'NONE', ( #3162 ), #1274, .T. ) ;
#4737=EDGE_CURVE ( 'NONE', #4838, #3126, #3995, .T. ) ;
#4740=CIRCLE ( 'NONE', #3613, 1.000000000000000888 ) ;
#4755=CARTESIAN_POINT ( 'NONE',  ( 0.000000000000000000, 0.000000000000000000, -32.00000000000000000 ) ) ;
#4773=EDGE_LOOP ( 'NONE', ( #1472, #1864 ) ) ;
#4779=DIRECTION ( 'NONE',  ( 1.000000000000000000, -0.000000000000000000, -0.000000000000000000 ) ) ;
#4781=CARTESIAN_POINT ( 'NONE',  ( 15.00000000000000000, 20.00000000000000355, -32.00000000000000000 ) ) ;
#4784=ORIENTED_EDGE ( 'NONE', *, *, #1703, .T. ) ;
#4801=CARTESIAN_POINT ( 'NONE',  ( 22.30741055306794962, -11.28818263778243924, -32.00000000000004263 ) ) ;
#4804=CARTESIAN_POINT ( 'NONE',  ( 15.00000000000000000, 16.00000000000000000, -20.00000000000000000 ) ) ;
#4812=ADVANCED_FACE ( 'NONE', ( #3575 ), #3206, .T. ) ;
#4815=DIRECTION ( 'NONE',  ( 0.000000000000000000, 0.000000000000000000, 1.000000000000000000 ) ) ;
#4817=AXIS2_PLACEMENT_3D ( 'NONE', #2257, #4475, #4127 ) ;
#4830=EDGE_CURVE ( 'NONE', #3603, #4310, #3185, .T. ) ;
#4834=DIRECTION ( 'NONE',  ( 1.000000000000000000, 0.000000000000000000, 0.000000000000000000 ) ) ;
#4836=CARTESIAN_POINT ( 'NONE',  ( 22.76747806470417856, -10.32821797429374833, -27.99768719324571364 ) ) ;
#4837=VECTOR ( 'NONE', #1164, 1000.000000000000000 ) ;
#4838=VERTEX_POINT ( 'NONE', #4490 ) ;
#4839=CARTESIAN_POINT ( 'NONE',  ( 22.47483654244695472, 10.94974330264383511, -22.75458106415069182 ) ) ;
#4841=CARTESIAN_POINT ( 'NONE',  ( 0.000000000000000000, 0.000000000000000000, -32.00000000000000000 ) ) ;
#4846=DIRECTION ( 'NONE',  ( 0.000000000000000000, 0.000000000000000000, -1.000000000000000000 ) ) ;
#4849=VERTEX_POINT ( 'NONE', #4873 ) ;
#4865=EDGE_LOOP ( 'NONE', ( #3499, #4898, #1535, #3118 ) ) ;
#4866=VERTEX_POINT ( 'NONE', #4440 ) ;
#4873=CARTESIAN_POINT ( 'NONE',  ( 15.00000000000000178, -16.00000000000000000, -23.35000000000001563 ) ) ;
#4879=AXIS2_PLACEMENT_3D ( 'NONE', #3369, #668, #294 ) ;
#4886=EDGE_CURVE ( 'NONE', #4359, #2811, #4065, .T. ) ;
#4898=ORIENTED_EDGE ( 'NONE', *, *, #489, .T. ) ;
#4901=CARTESIAN_POINT ( 'NONE',  ( 2.444036937190193033E-14, 6.999999999999999112, -32.00000000000000000 ) ) ;
#4909=DIRECTION ( 'NONE',  ( 0.000000000000000000, 0.000000000000000000, -1.000000000000000000 ) ) ;
#4910=ORIENTED_EDGE ( 'NONE', *, *, #2627, .F. ) ;
#4917=ORIENTED_EDGE ( 'NONE', *, *, #1242, .F. ) ;
#4919=ADVANCED_FACE ( 'NONE', ( #4043, #2571 ), #2222, .T. ) ;
#4920=ADVANCED_FACE ( 'NONE', ( #3302 ), #1817, .F. ) ;
#4922=EDGE_LOOP ( 'NONE', ( #273, #1813, #2224, #4126 ) ) ;
#4932=( LENGTH_UNIT ( ) NAMED_UNIT ( * ) SI_UNIT ( .MILLI., .METRE. ) );
#4939=CARTESIAN_POINT ( 'NONE',  ( 2.444036937190193033E-14, 6.999999999999999112, -20.00000000000000000 ) ) ;
#4948=CARTESIAN_POINT ( 'NONE',  ( 15.00000000000000000, 16.00000000000000000, -32.00000000000000000 ) ) ;
#4958=LINE ( 'NONE', #2629, #924 ) ;
ENDSEC;
END-ISO-10303-21;
